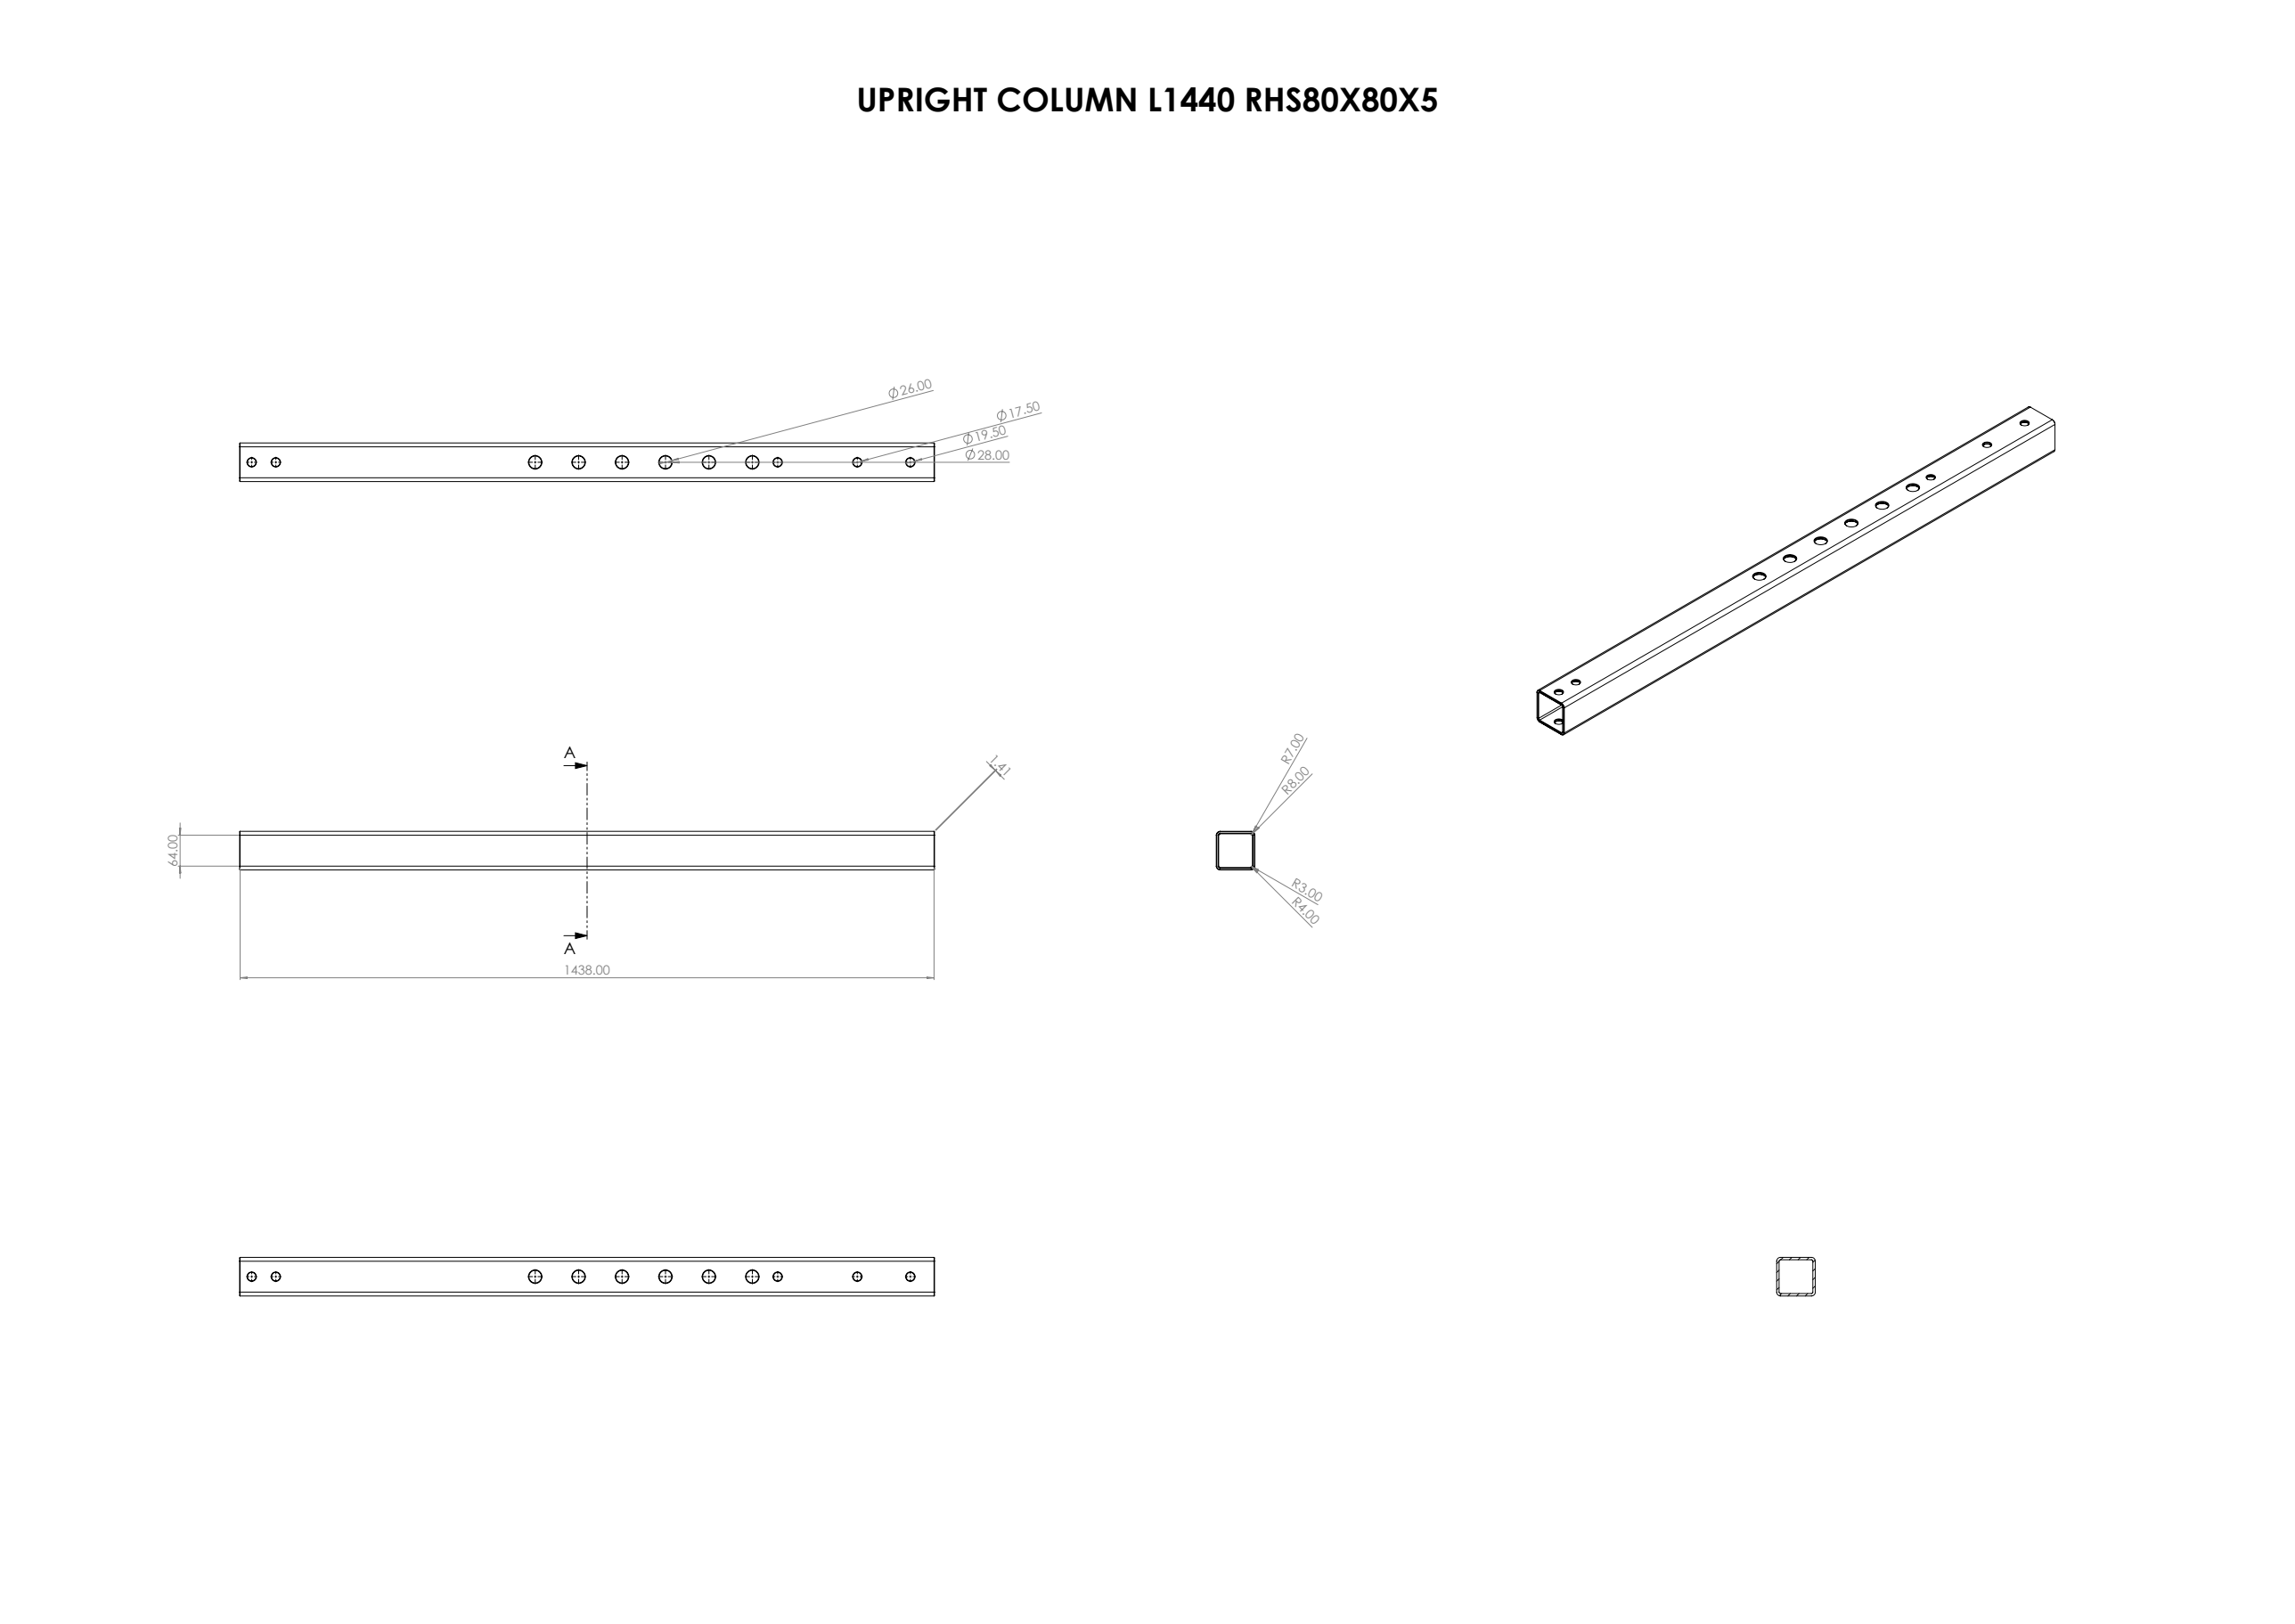
ISO-10303-21;
HEADER;
/* Generated by software containing ST-Developer
 * from STEP Tools, Inc. (www.steptools.com) 
 */

FILE_DESCRIPTION(
/* description */ (''),
/* implementation_level */ '2;1');

FILE_NAME(
/* name */ '01_Upright_Column_L1440_RHS80x80x5.step',
/* time_stamp */ '2026-10-20T10:03:03-07:00',
/* author */ (''),
/* organization */ (''),
/* preprocessor_version */ 'ST-DEVELOPER v20.2',
/* originating_system */ 'Autodesk Translation Framework v15.15.0.0',
/* authorisation */ '');

FILE_SCHEMA (('AUTOMOTIVE_DESIGN { 1 0 10303 214 3 1 1 }'));
ENDSEC;

DATA;
#10=MECHANICAL_DESIGN_GEOMETRIC_PRESENTATION_REPRESENTATION('',(#550),#71492);
#400=SHAPE_REPRESENTATION_RELATIONSHIP('SRR','None',#71621,#419);
#419=ADVANCED_BREP_SHAPE_REPRESENTATION('',(#438),#71491);
#438=MANIFOLD_SOLID_BREP('Upright',#28477);
#550=STYLED_ITEM('',(#71873),#438);
#1844=CYLINDRICAL_SURFACE('',#30568,0.875);
#1845=CYLINDRICAL_SURFACE('',#30572,0.875);
#1846=CYLINDRICAL_SURFACE('',#30576,0.875);
#1847=CYLINDRICAL_SURFACE('',#30580,0.875);
#1848=CYLINDRICAL_SURFACE('',#30584,0.875);
#1849=CYLINDRICAL_SURFACE('',#30588,1.3);
#1850=CYLINDRICAL_SURFACE('',#30592,1.3);
#1851=CYLINDRICAL_SURFACE('',#30608,0.875);
#1852=CYLINDRICAL_SURFACE('',#30612,0.875);
#1853=CYLINDRICAL_SURFACE('',#30616,0.875);
#1854=CYLINDRICAL_SURFACE('',#30620,0.875);
#1855=CYLINDRICAL_SURFACE('',#30624,0.875);
#1856=CYLINDRICAL_SURFACE('',#30642,0.3);
#1857=CYLINDRICAL_SURFACE('',#30645,0.3);
#1858=CYLINDRICAL_SURFACE('',#30654,1.3);
#1859=CYLINDRICAL_SURFACE('',#30658,1.3);
#1860=CYLINDRICAL_SURFACE('',#30662,1.3);
#1861=CYLINDRICAL_SURFACE('',#30666,1.3);
#1862=CYLINDRICAL_SURFACE('',#30670,1.3);
#1863=CYLINDRICAL_SURFACE('',#30674,1.3);
#1864=CYLINDRICAL_SURFACE('',#30678,1.3);
#1865=CYLINDRICAL_SURFACE('',#30682,1.3);
#1866=CYLINDRICAL_SURFACE('',#30686,1.3);
#1867=CYLINDRICAL_SURFACE('',#30707,1.3);
#1868=CYLINDRICAL_SURFACE('',#30738,0.8);
#1869=CYLINDRICAL_SURFACE('',#30741,0.8);
#1870=CYLINDRICAL_SURFACE('',#30769,0.8);
#1871=CYLINDRICAL_SURFACE('',#30785,0.3);
#1872=CYLINDRICAL_SURFACE('',#30786,0.3);
#1873=CYLINDRICAL_SURFACE('',#30789,0.8);
#1999=FACE_BOUND('',#6142,.T.);
#2000=FACE_BOUND('',#6143,.T.);
#2001=FACE_BOUND('',#6144,.T.);
#2002=FACE_BOUND('',#6145,.T.);
#2003=FACE_BOUND('',#6146,.T.);
#2004=FACE_BOUND('',#6147,.T.);
#2005=FACE_BOUND('',#6148,.T.);
#2006=FACE_BOUND('',#6149,.T.);
#2007=FACE_BOUND('',#6150,.T.);
#2008=FACE_BOUND('',#6151,.T.);
#2009=FACE_BOUND('',#6152,.T.);
#2010=FACE_BOUND('',#6168,.T.);
#2011=FACE_BOUND('',#6169,.T.);
#2012=FACE_BOUND('',#6170,.T.);
#2013=FACE_BOUND('',#6171,.T.);
#2014=FACE_BOUND('',#6172,.T.);
#2015=FACE_BOUND('',#6173,.T.);
#2016=FACE_BOUND('',#6174,.T.);
#2017=FACE_BOUND('',#6175,.T.);
#2018=FACE_BOUND('',#6176,.T.);
#2019=FACE_BOUND('',#6177,.T.);
#2020=FACE_BOUND('',#6178,.T.);
#2021=FACE_BOUND('',#6200,.T.);
#2022=FACE_BOUND('',#6221,.T.);
#2023=FACE_BOUND('',#6222,.T.);
#2024=FACE_BOUND('',#6223,.T.);
#2025=FACE_BOUND('',#6224,.T.);
#2026=FACE_BOUND('',#6225,.T.);
#2027=FACE_BOUND('',#6226,.T.);
#2028=FACE_BOUND('',#6227,.T.);
#2029=FACE_BOUND('',#6228,.T.);
#2030=FACE_BOUND('',#6229,.T.);
#2031=FACE_BOUND('',#6230,.T.);
#2032=FACE_BOUND('',#6231,.T.);
#2033=FACE_BOUND('',#6240,.T.);
#2034=FACE_BOUND('',#6241,.T.);
#2035=FACE_BOUND('',#6242,.T.);
#2036=FACE_BOUND('',#6243,.T.);
#2037=FACE_BOUND('',#6244,.T.);
#2038=FACE_BOUND('',#6245,.T.);
#2039=FACE_BOUND('',#6246,.T.);
#2040=FACE_BOUND('',#6247,.T.);
#2041=FACE_BOUND('',#6248,.T.);
#2042=FACE_BOUND('',#6249,.T.);
#2043=FACE_BOUND('',#6250,.T.);
#2044=FACE_BOUND('',#6288,.T.);
#2611=CIRCLE('',#30555,0.975000000000001);
#2612=CIRCLE('',#30556,0.875);
#2613=CIRCLE('',#30558,0.975000000000001);
#2614=CIRCLE('',#30559,0.975000000000001);
#2615=CIRCLE('',#30560,1.4);
#2616=CIRCLE('',#30561,1.4);
#2617=CIRCLE('',#30562,1.4);
#2618=CIRCLE('',#30563,1.4);
#2619=CIRCLE('',#30564,1.4);
#2620=CIRCLE('',#30565,1.4);
#2621=CIRCLE('',#30566,0.975000000000001);
#2622=CIRCLE('',#30567,0.975000000000001);
#2623=CIRCLE('',#30569,0.875);
#2624=CIRCLE('',#30571,0.875);
#2625=CIRCLE('',#30573,0.875);
#2626=CIRCLE('',#30575,0.875);
#2627=CIRCLE('',#30577,0.875);
#2628=CIRCLE('',#30579,0.875);
#2629=CIRCLE('',#30581,0.875);
#2630=CIRCLE('',#30583,0.875);
#2631=CIRCLE('',#30585,0.875);
#2632=CIRCLE('',#30587,1.3);
#2633=CIRCLE('',#30589,1.3);
#2634=CIRCLE('',#30591,1.3);
#2635=CIRCLE('',#30593,1.3);
#2636=CIRCLE('',#30595,0.975000000000001);
#2637=CIRCLE('',#30596,0.875);
#2638=CIRCLE('',#30598,0.975000000000001);
#2639=CIRCLE('',#30599,0.975000000000001);
#2640=CIRCLE('',#30600,1.4);
#2641=CIRCLE('',#30601,1.4);
#2642=CIRCLE('',#30602,1.4);
#2643=CIRCLE('',#30603,1.4);
#2644=CIRCLE('',#30604,1.4);
#2645=CIRCLE('',#30605,1.4);
#2646=CIRCLE('',#30606,0.975000000000001);
#2647=CIRCLE('',#30607,0.975000000000001);
#2648=CIRCLE('',#30609,0.875);
#2649=CIRCLE('',#30611,0.875);
#2650=CIRCLE('',#30613,0.875);
#2651=CIRCLE('',#30615,0.875);
#2652=CIRCLE('',#30617,0.875);
#2653=CIRCLE('',#30619,0.875);
#2654=CIRCLE('',#30621,0.875);
#2655=CIRCLE('',#30623,0.875);
#2656=CIRCLE('',#30625,0.875);
#2657=CIRCLE('',#30628,0.3);
#2658=CIRCLE('',#30629,0.400000000000004);
#2659=CIRCLE('',#30632,0.3);
#2660=CIRCLE('',#30633,0.4);
#2661=CIRCLE('',#30636,0.3);
#2662=CIRCLE('',#30637,0.400000000000003);
#2663=CIRCLE('',#30640,0.3);
#2664=CIRCLE('',#30641,0.400000000000003);
#2665=CIRCLE('',#30643,0.3);
#2666=CIRCLE('',#30646,0.3);
#2667=CIRCLE('',#30648,0.699999999999997);
#2668=CIRCLE('',#30649,0.699999999999997);
#2669=CIRCLE('',#30650,0.7);
#2670=CIRCLE('',#30651,0.700000000000001);
#2671=CIRCLE('',#30653,1.3);
#2672=CIRCLE('',#30655,1.3);
#2673=CIRCLE('',#30657,1.3);
#2674=CIRCLE('',#30659,1.3);
#2675=CIRCLE('',#30661,1.3);
#2676=CIRCLE('',#30663,1.3);
#2677=CIRCLE('',#30665,1.3);
#2678=CIRCLE('',#30667,1.3);
#2679=CIRCLE('',#30669,1.3);
#2680=CIRCLE('',#30671,1.3);
#2681=CIRCLE('',#30673,1.3);
#2682=CIRCLE('',#30675,1.3);
#2683=CIRCLE('',#30677,1.3);
#2684=CIRCLE('',#30679,1.3);
#2685=CIRCLE('',#30681,1.3);
#2686=CIRCLE('',#30683,1.3);
#2687=CIRCLE('',#30685,1.3);
#2688=CIRCLE('',#30687,1.3);
#2689=CIRCLE('',#30689,0.975000000000001);
#2690=CIRCLE('',#30691,0.975000000000001);
#2691=CIRCLE('',#30692,0.975000000000001);
#2692=CIRCLE('',#30693,1.4);
#2693=CIRCLE('',#30694,1.4);
#2694=CIRCLE('',#30695,1.4);
#2695=CIRCLE('',#30696,1.4);
#2696=CIRCLE('',#30697,1.4);
#2697=CIRCLE('',#30698,1.4);
#2698=CIRCLE('',#30699,0.975000000000001);
#2699=CIRCLE('',#30700,0.975000000000001);
#2700=CIRCLE('',#30706,1.3);
#2701=CIRCLE('',#30708,1.3);
#2702=CIRCLE('',#30710,0.975000000000001);
#2703=CIRCLE('',#30712,0.975000000000001);
#2704=CIRCLE('',#30713,0.975000000000001);
#2705=CIRCLE('',#30714,1.4);
#2706=CIRCLE('',#30715,1.4);
#2707=CIRCLE('',#30716,1.4);
#2708=CIRCLE('',#30717,1.4);
#2709=CIRCLE('',#30718,1.4);
#2710=CIRCLE('',#30719,1.4);
#2711=CIRCLE('',#30720,0.975000000000001);
#2712=CIRCLE('',#30721,0.975000000000001);
#2713=CIRCLE('',#30728,0.8);
#2714=CIRCLE('',#30731,0.8);
#2715=CIRCLE('',#30734,0.8);
#2716=CIRCLE('',#30737,0.8);
#2717=CIRCLE('',#30739,0.8);
#2718=CIRCLE('',#30742,0.8);
#2719=CIRCLE('',#30756,0.8);
#2720=CIRCLE('',#30757,0.7);
#2721=CIRCLE('',#30760,0.8);
#2722=CIRCLE('',#30761,0.700000000000001);
#2723=CIRCLE('',#30764,0.699999999999997);
#2724=CIRCLE('',#30767,0.699999999999997);
#2725=CIRCLE('',#30771,0.4);
#2726=CIRCLE('',#30772,0.400000000000003);
#2727=CIRCLE('',#30773,0.400000000000003);
#2728=CIRCLE('',#30774,0.400000000000004);
#2729=CIRCLE('',#30776,0.3);
#2730=CIRCLE('',#30779,0.3);
#2911=CONICAL_SURFACE('',#30554,0.925000000000001,0.785398163397455);
#2912=CONICAL_SURFACE('',#30570,0.925000000000001,0.785398163397455);
#2913=CONICAL_SURFACE('',#30574,0.925000000000001,0.785398163397455);
#2914=CONICAL_SURFACE('',#30578,0.925000000000001,0.785398163397455);
#2915=CONICAL_SURFACE('',#30582,0.925000000000001,0.785398163397455);
#2916=CONICAL_SURFACE('',#30586,1.35,0.785398163397455);
#2917=CONICAL_SURFACE('',#30590,1.35,0.785398163397455);
#2918=CONICAL_SURFACE('',#30594,0.925000000000001,0.785398163397455);
#2919=CONICAL_SURFACE('',#30610,0.925000000000001,0.785398163397455);
#2920=CONICAL_SURFACE('',#30614,0.925000000000001,0.785398163397455);
#2921=CONICAL_SURFACE('',#30618,0.925000000000001,0.785398163397455);
#2922=CONICAL_SURFACE('',#30622,0.925000000000001,0.785398163397455);
#2923=CONICAL_SURFACE('',#30627,0.350000000000002,0.785398163397469);
#2924=CONICAL_SURFACE('',#30631,0.35,0.785398163397446);
#2925=CONICAL_SURFACE('',#30635,0.350000000000001,0.785398163397461);
#2926=CONICAL_SURFACE('',#30639,0.350000000000001,0.785398163397461);
#2927=CONICAL_SURFACE('',#30652,1.35,0.785398163397455);
#2928=CONICAL_SURFACE('',#30656,1.35,0.785398163397455);
#2929=CONICAL_SURFACE('',#30660,1.35,0.785398163397455);
#2930=CONICAL_SURFACE('',#30664,1.35,0.785398163397455);
#2931=CONICAL_SURFACE('',#30668,1.35,0.785398163397455);
#2932=CONICAL_SURFACE('',#30672,1.35,0.785398163397455);
#2933=CONICAL_SURFACE('',#30676,1.35,0.785398163397455);
#2934=CONICAL_SURFACE('',#30680,1.35,0.785398163397455);
#2935=CONICAL_SURFACE('',#30684,1.35,0.785398163397455);
#2936=CONICAL_SURFACE('',#30688,0.925000000000001,0.785398163397455);
#2937=CONICAL_SURFACE('',#30701,0.925000000000001,0.785398163397455);
#2938=CONICAL_SURFACE('',#30702,0.925000000000001,0.785398163397455);
#2939=CONICAL_SURFACE('',#30703,0.925000000000001,0.785398163397455);
#2940=CONICAL_SURFACE('',#30704,0.925000000000001,0.785398163397455);
#2941=CONICAL_SURFACE('',#30705,1.35,0.785398163397455);
#2942=CONICAL_SURFACE('',#30709,0.925000000000001,0.785398163397455);
#2943=CONICAL_SURFACE('',#30722,0.925000000000001,0.785398163397455);
#2944=CONICAL_SURFACE('',#30723,0.925000000000001,0.785398163397455);
#2945=CONICAL_SURFACE('',#30724,0.925000000000001,0.785398163397455);
#2946=CONICAL_SURFACE('',#30725,0.925000000000001,0.785398163397455);
#2947=CONICAL_SURFACE('',#30727,0.75,0.785398163397444);
#2948=CONICAL_SURFACE('',#30730,0.75,0.785398163397447);
#2949=CONICAL_SURFACE('',#30733,0.749999999999998,0.785398163397465);
#2950=CONICAL_SURFACE('',#30736,0.749999999999998,0.785398163397465);
#2951=CONICAL_SURFACE('',#30743,1.35,0.785398163397455);
#2952=CONICAL_SURFACE('',#30744,1.35,0.785398163397455);
#2953=CONICAL_SURFACE('',#30745,1.35,0.785398163397455);
#2954=CONICAL_SURFACE('',#30746,1.35,0.785398163397455);
#2955=CONICAL_SURFACE('',#30747,1.35,0.785398163397455);
#2956=CONICAL_SURFACE('',#30748,1.35,0.785398163397455);
#2957=CONICAL_SURFACE('',#30749,1.35,0.785398163397455);
#2958=CONICAL_SURFACE('',#30750,1.35,0.785398163397455);
#2959=CONICAL_SURFACE('',#30751,1.35,0.785398163397455);
#2960=CONICAL_SURFACE('',#30752,1.35,0.785398163397455);
#2961=CONICAL_SURFACE('',#30753,1.35,0.785398163397455);
#2962=CONICAL_SURFACE('',#30754,1.35,0.785398163397455);
#2963=CONICAL_SURFACE('',#30755,0.75,0.785398163397475);
#2964=CONICAL_SURFACE('',#30759,0.75,0.785398163397472);
#2965=CONICAL_SURFACE('',#30763,0.749999999999998,0.785398163397494);
#2966=CONICAL_SURFACE('',#30766,0.749999999999998,0.785398163397494);
#2967=CONICAL_SURFACE('',#30775,0.35,0.785398163397474);
#2968=CONICAL_SURFACE('',#30778,0.350000000000002,0.785398163397498);
#2969=CONICAL_SURFACE('',#30781,0.350000000000001,0.78539816339749);
#2970=CONICAL_SURFACE('',#30783,0.350000000000001,0.78539816339749);
#4435=FACE_OUTER_BOUND('',#6140,.T.);
#4436=FACE_OUTER_BOUND('',#6141,.T.);
#4437=FACE_OUTER_BOUND('',#6153,.T.);
#4438=FACE_OUTER_BOUND('',#6154,.T.);
#4439=FACE_OUTER_BOUND('',#6155,.T.);
#4440=FACE_OUTER_BOUND('',#6156,.T.);
#4441=FACE_OUTER_BOUND('',#6157,.T.);
#4442=FACE_OUTER_BOUND('',#6158,.T.);
#4443=FACE_OUTER_BOUND('',#6159,.T.);
#4444=FACE_OUTER_BOUND('',#6160,.T.);
#4445=FACE_OUTER_BOUND('',#6161,.T.);
#4446=FACE_OUTER_BOUND('',#6162,.T.);
#4447=FACE_OUTER_BOUND('',#6163,.T.);
#4448=FACE_OUTER_BOUND('',#6164,.T.);
#4449=FACE_OUTER_BOUND('',#6165,.T.);
#4450=FACE_OUTER_BOUND('',#6166,.T.);
#4451=FACE_OUTER_BOUND('',#6167,.T.);
#4452=FACE_OUTER_BOUND('',#6179,.T.);
#4453=FACE_OUTER_BOUND('',#6180,.T.);
#4454=FACE_OUTER_BOUND('',#6181,.T.);
#4455=FACE_OUTER_BOUND('',#6182,.T.);
#4456=FACE_OUTER_BOUND('',#6183,.T.);
#4457=FACE_OUTER_BOUND('',#6184,.T.);
#4458=FACE_OUTER_BOUND('',#6185,.T.);
#4459=FACE_OUTER_BOUND('',#6186,.T.);
#4460=FACE_OUTER_BOUND('',#6187,.T.);
#4461=FACE_OUTER_BOUND('',#6188,.T.);
#4462=FACE_OUTER_BOUND('',#6189,.T.);
#4463=FACE_OUTER_BOUND('',#6190,.T.);
#4464=FACE_OUTER_BOUND('',#6191,.T.);
#4465=FACE_OUTER_BOUND('',#6192,.T.);
#4466=FACE_OUTER_BOUND('',#6193,.T.);
#4467=FACE_OUTER_BOUND('',#6194,.T.);
#4468=FACE_OUTER_BOUND('',#6195,.T.);
#4469=FACE_OUTER_BOUND('',#6196,.T.);
#4470=FACE_OUTER_BOUND('',#6197,.T.);
#4471=FACE_OUTER_BOUND('',#6198,.T.);
#4472=FACE_OUTER_BOUND('',#6199,.T.);
#4473=FACE_OUTER_BOUND('',#6201,.T.);
#4474=FACE_OUTER_BOUND('',#6202,.T.);
#4475=FACE_OUTER_BOUND('',#6203,.T.);
#4476=FACE_OUTER_BOUND('',#6204,.T.);
#4477=FACE_OUTER_BOUND('',#6205,.T.);
#4478=FACE_OUTER_BOUND('',#6206,.T.);
#4479=FACE_OUTER_BOUND('',#6207,.T.);
#4480=FACE_OUTER_BOUND('',#6208,.T.);
#4481=FACE_OUTER_BOUND('',#6209,.T.);
#4482=FACE_OUTER_BOUND('',#6210,.T.);
#4483=FACE_OUTER_BOUND('',#6211,.T.);
#4484=FACE_OUTER_BOUND('',#6212,.T.);
#4485=FACE_OUTER_BOUND('',#6213,.T.);
#4486=FACE_OUTER_BOUND('',#6214,.T.);
#4487=FACE_OUTER_BOUND('',#6215,.T.);
#4488=FACE_OUTER_BOUND('',#6216,.T.);
#4489=FACE_OUTER_BOUND('',#6217,.T.);
#4490=FACE_OUTER_BOUND('',#6218,.T.);
#4491=FACE_OUTER_BOUND('',#6219,.T.);
#4492=FACE_OUTER_BOUND('',#6220,.T.);
#4493=FACE_OUTER_BOUND('',#6232,.T.);
#4494=FACE_OUTER_BOUND('',#6233,.T.);
#4495=FACE_OUTER_BOUND('',#6234,.T.);
#4496=FACE_OUTER_BOUND('',#6235,.T.);
#4497=FACE_OUTER_BOUND('',#6236,.T.);
#4498=FACE_OUTER_BOUND('',#6237,.T.);
#4499=FACE_OUTER_BOUND('',#6238,.T.);
#4500=FACE_OUTER_BOUND('',#6239,.T.);
#4501=FACE_OUTER_BOUND('',#6251,.T.);
#4502=FACE_OUTER_BOUND('',#6252,.T.);
#4503=FACE_OUTER_BOUND('',#6253,.T.);
#4504=FACE_OUTER_BOUND('',#6254,.T.);
#4505=FACE_OUTER_BOUND('',#6255,.T.);
#4506=FACE_OUTER_BOUND('',#6256,.T.);
#4507=FACE_OUTER_BOUND('',#6257,.T.);
#4508=FACE_OUTER_BOUND('',#6258,.T.);
#4509=FACE_OUTER_BOUND('',#6259,.T.);
#4510=FACE_OUTER_BOUND('',#6260,.T.);
#4511=FACE_OUTER_BOUND('',#6261,.T.);
#4512=FACE_OUTER_BOUND('',#6262,.T.);
#4513=FACE_OUTER_BOUND('',#6263,.T.);
#4514=FACE_OUTER_BOUND('',#6264,.T.);
#4515=FACE_OUTER_BOUND('',#6265,.T.);
#4516=FACE_OUTER_BOUND('',#6266,.T.);
#4517=FACE_OUTER_BOUND('',#6267,.T.);
#4518=FACE_OUTER_BOUND('',#6268,.T.);
#4519=FACE_OUTER_BOUND('',#6269,.T.);
#4520=FACE_OUTER_BOUND('',#6270,.T.);
#4521=FACE_OUTER_BOUND('',#6271,.T.);
#4522=FACE_OUTER_BOUND('',#6272,.T.);
#4523=FACE_OUTER_BOUND('',#6273,.T.);
#4524=FACE_OUTER_BOUND('',#6274,.T.);
#4525=FACE_OUTER_BOUND('',#6275,.T.);
#4526=FACE_OUTER_BOUND('',#6276,.T.);
#4527=FACE_OUTER_BOUND('',#6277,.T.);
#4528=FACE_OUTER_BOUND('',#6278,.T.);
#4529=FACE_OUTER_BOUND('',#6279,.T.);
#4530=FACE_OUTER_BOUND('',#6280,.T.);
#4531=FACE_OUTER_BOUND('',#6281,.T.);
#4532=FACE_OUTER_BOUND('',#6282,.T.);
#4533=FACE_OUTER_BOUND('',#6283,.T.);
#4534=FACE_OUTER_BOUND('',#6284,.T.);
#4535=FACE_OUTER_BOUND('',#6285,.T.);
#4536=FACE_OUTER_BOUND('',#6286,.T.);
#4537=FACE_OUTER_BOUND('',#6287,.T.);
#4538=FACE_OUTER_BOUND('',#6289,.T.);
#4539=FACE_OUTER_BOUND('',#6290,.T.);
#4540=FACE_OUTER_BOUND('',#6291,.T.);
#4541=FACE_OUTER_BOUND('',#6292,.T.);
#4542=FACE_OUTER_BOUND('',#6293,.T.);
#4543=FACE_OUTER_BOUND('',#6294,.T.);
#4544=FACE_OUTER_BOUND('',#6295,.T.);
#4545=FACE_OUTER_BOUND('',#6296,.T.);
#4546=FACE_OUTER_BOUND('',#6297,.T.);
#4547=FACE_OUTER_BOUND('',#6298,.T.);
#4548=FACE_OUTER_BOUND('',#6299,.T.);
#4549=FACE_OUTER_BOUND('',#6300,.T.);
#4550=FACE_OUTER_BOUND('',#6301,.T.);
#6140=EDGE_LOOP('',(#25539,#25540,#25541,#25542));
#6141=EDGE_LOOP('',(#25543,#25544,#25545,#25546));
#6142=EDGE_LOOP('',(#25547));
#6143=EDGE_LOOP('',(#25548));
#6144=EDGE_LOOP('',(#25549));
#6145=EDGE_LOOP('',(#25550));
#6146=EDGE_LOOP('',(#25551));
#6147=EDGE_LOOP('',(#25552));
#6148=EDGE_LOOP('',(#25553));
#6149=EDGE_LOOP('',(#25554));
#6150=EDGE_LOOP('',(#25555));
#6151=EDGE_LOOP('',(#25556));
#6152=EDGE_LOOP('',(#25557));
#6153=EDGE_LOOP('',(#25558,#25559,#25560,#25561));
#6154=EDGE_LOOP('',(#25562,#25563,#25564,#25565));
#6155=EDGE_LOOP('',(#25566,#25567,#25568,#25569));
#6156=EDGE_LOOP('',(#25570,#25571,#25572,#25573));
#6157=EDGE_LOOP('',(#25574,#25575,#25576,#25577));
#6158=EDGE_LOOP('',(#25578,#25579,#25580,#25581));
#6159=EDGE_LOOP('',(#25582,#25583,#25584,#25585));
#6160=EDGE_LOOP('',(#25586,#25587,#25588,#25589));
#6161=EDGE_LOOP('',(#25590,#25591,#25592,#25593));
#6162=EDGE_LOOP('',(#25594,#25595,#25596,#25597));
#6163=EDGE_LOOP('',(#25598,#25599,#25600,#25601));
#6164=EDGE_LOOP('',(#25602,#25603,#25604,#25605));
#6165=EDGE_LOOP('',(#25606,#25607,#25608,#25609));
#6166=EDGE_LOOP('',(#25610,#25611,#25612,#25613));
#6167=EDGE_LOOP('',(#25614,#25615,#25616,#25617));
#6168=EDGE_LOOP('',(#25618));
#6169=EDGE_LOOP('',(#25619));
#6170=EDGE_LOOP('',(#25620));
#6171=EDGE_LOOP('',(#25621));
#6172=EDGE_LOOP('',(#25622));
#6173=EDGE_LOOP('',(#25623));
#6174=EDGE_LOOP('',(#25624));
#6175=EDGE_LOOP('',(#25625));
#6176=EDGE_LOOP('',(#25626));
#6177=EDGE_LOOP('',(#25627));
#6178=EDGE_LOOP('',(#25628));
#6179=EDGE_LOOP('',(#25629,#25630,#25631,#25632));
#6180=EDGE_LOOP('',(#25633,#25634,#25635,#25636));
#6181=EDGE_LOOP('',(#25637,#25638,#25639,#25640));
#6182=EDGE_LOOP('',(#25641,#25642,#25643,#25644));
#6183=EDGE_LOOP('',(#25645,#25646,#25647,#25648));
#6184=EDGE_LOOP('',(#25649,#25650,#25651,#25652));
#6185=EDGE_LOOP('',(#25653,#25654,#25655,#25656));
#6186=EDGE_LOOP('',(#25657,#25658,#25659,#25660));
#6187=EDGE_LOOP('',(#25661,#25662,#25663,#25664));
#6188=EDGE_LOOP('',(#25665,#25666,#25667,#25668));
#6189=EDGE_LOOP('',(#25669,#25670,#25671,#25672));
#6190=EDGE_LOOP('',(#25673,#25674,#25675,#25676));
#6191=EDGE_LOOP('',(#25677,#25678,#25679,#25680));
#6192=EDGE_LOOP('',(#25681,#25682,#25683,#25684));
#6193=EDGE_LOOP('',(#25685,#25686,#25687,#25688));
#6194=EDGE_LOOP('',(#25689,#25690,#25691,#25692));
#6195=EDGE_LOOP('',(#25693,#25694,#25695,#25696));
#6196=EDGE_LOOP('',(#25697,#25698,#25699,#25700));
#6197=EDGE_LOOP('',(#25701,#25702,#25703,#25704));
#6198=EDGE_LOOP('',(#25705,#25706,#25707,#25708));
#6199=EDGE_LOOP('',(#25709,#25710,#25711,#25712,#25713,#25714,#25715,#25716));
#6200=EDGE_LOOP('',(#25717,#25718,#25719,#25720,#25721,#25722,#25723,#25724));
#6201=EDGE_LOOP('',(#25725,#25726,#25727,#25728));
#6202=EDGE_LOOP('',(#25729,#25730,#25731,#25732));
#6203=EDGE_LOOP('',(#25733,#25734,#25735,#25736));
#6204=EDGE_LOOP('',(#25737,#25738,#25739,#25740));
#6205=EDGE_LOOP('',(#25741,#25742,#25743,#25744));
#6206=EDGE_LOOP('',(#25745,#25746,#25747,#25748));
#6207=EDGE_LOOP('',(#25749,#25750,#25751,#25752));
#6208=EDGE_LOOP('',(#25753,#25754,#25755,#25756));
#6209=EDGE_LOOP('',(#25757,#25758,#25759,#25760));
#6210=EDGE_LOOP('',(#25761,#25762,#25763,#25764));
#6211=EDGE_LOOP('',(#25765,#25766,#25767,#25768));
#6212=EDGE_LOOP('',(#25769,#25770,#25771,#25772));
#6213=EDGE_LOOP('',(#25773,#25774,#25775,#25776));
#6214=EDGE_LOOP('',(#25777,#25778,#25779,#25780));
#6215=EDGE_LOOP('',(#25781,#25782,#25783,#25784));
#6216=EDGE_LOOP('',(#25785,#25786,#25787,#25788));
#6217=EDGE_LOOP('',(#25789,#25790,#25791,#25792));
#6218=EDGE_LOOP('',(#25793,#25794,#25795,#25796));
#6219=EDGE_LOOP('',(#25797,#25798,#25799,#25800));
#6220=EDGE_LOOP('',(#25801,#25802,#25803,#25804));
#6221=EDGE_LOOP('',(#25805));
#6222=EDGE_LOOP('',(#25806));
#6223=EDGE_LOOP('',(#25807));
#6224=EDGE_LOOP('',(#25808));
#6225=EDGE_LOOP('',(#25809));
#6226=EDGE_LOOP('',(#25810));
#6227=EDGE_LOOP('',(#25811));
#6228=EDGE_LOOP('',(#25812));
#6229=EDGE_LOOP('',(#25813));
#6230=EDGE_LOOP('',(#25814));
#6231=EDGE_LOOP('',(#25815));
#6232=EDGE_LOOP('',(#25816,#25817,#25818,#25819));
#6233=EDGE_LOOP('',(#25820,#25821,#25822,#25823));
#6234=EDGE_LOOP('',(#25824,#25825,#25826,#25827));
#6235=EDGE_LOOP('',(#25828,#25829,#25830,#25831));
#6236=EDGE_LOOP('',(#25832,#25833,#25834,#25835));
#6237=EDGE_LOOP('',(#25836,#25837,#25838,#25839));
#6238=EDGE_LOOP('',(#25840,#25841,#25842,#25843));
#6239=EDGE_LOOP('',(#25844,#25845,#25846,#25847));
#6240=EDGE_LOOP('',(#25848));
#6241=EDGE_LOOP('',(#25849));
#6242=EDGE_LOOP('',(#25850));
#6243=EDGE_LOOP('',(#25851));
#6244=EDGE_LOOP('',(#25852));
#6245=EDGE_LOOP('',(#25853));
#6246=EDGE_LOOP('',(#25854));
#6247=EDGE_LOOP('',(#25855));
#6248=EDGE_LOOP('',(#25856));
#6249=EDGE_LOOP('',(#25857));
#6250=EDGE_LOOP('',(#25858));
#6251=EDGE_LOOP('',(#25859,#25860,#25861,#25862));
#6252=EDGE_LOOP('',(#25863,#25864,#25865,#25866));
#6253=EDGE_LOOP('',(#25867,#25868,#25869,#25870));
#6254=EDGE_LOOP('',(#25871,#25872,#25873,#25874));
#6255=EDGE_LOOP('',(#25875,#25876,#25877,#25878));
#6256=EDGE_LOOP('',(#25879,#25880,#25881,#25882));
#6257=EDGE_LOOP('',(#25883,#25884,#25885,#25886));
#6258=EDGE_LOOP('',(#25887,#25888,#25889,#25890));
#6259=EDGE_LOOP('',(#25891,#25892,#25893,#25894));
#6260=EDGE_LOOP('',(#25895,#25896,#25897,#25898));
#6261=EDGE_LOOP('',(#25899,#25900,#25901,#25902));
#6262=EDGE_LOOP('',(#25903,#25904,#25905,#25906));
#6263=EDGE_LOOP('',(#25907,#25908,#25909,#25910));
#6264=EDGE_LOOP('',(#25911,#25912,#25913,#25914));
#6265=EDGE_LOOP('',(#25915,#25916,#25917,#25918));
#6266=EDGE_LOOP('',(#25919,#25920,#25921,#25922));
#6267=EDGE_LOOP('',(#25923,#25924,#25925,#25926));
#6268=EDGE_LOOP('',(#25927,#25928,#25929,#25930));
#6269=EDGE_LOOP('',(#25931,#25932,#25933,#25934));
#6270=EDGE_LOOP('',(#25935,#25936,#25937,#25938));
#6271=EDGE_LOOP('',(#25939,#25940,#25941,#25942));
#6272=EDGE_LOOP('',(#25943,#25944,#25945,#25946));
#6273=EDGE_LOOP('',(#25947,#25948,#25949,#25950));
#6274=EDGE_LOOP('',(#25951,#25952,#25953,#25954));
#6275=EDGE_LOOP('',(#25955,#25956,#25957,#25958));
#6276=EDGE_LOOP('',(#25959,#25960,#25961,#25962));
#6277=EDGE_LOOP('',(#25963,#25964,#25965,#25966));
#6278=EDGE_LOOP('',(#25967,#25968,#25969,#25970));
#6279=EDGE_LOOP('',(#25971,#25972,#25973,#25974));
#6280=EDGE_LOOP('',(#25975,#25976,#25977,#25978));
#6281=EDGE_LOOP('',(#25979,#25980,#25981,#25982));
#6282=EDGE_LOOP('',(#25983,#25984,#25985,#25986));
#6283=EDGE_LOOP('',(#25987,#25988,#25989,#25990));
#6284=EDGE_LOOP('',(#25991,#25992,#25993,#25994));
#6285=EDGE_LOOP('',(#25995,#25996,#25997,#25998));
#6286=EDGE_LOOP('',(#25999,#26000,#26001,#26002));
#6287=EDGE_LOOP('',(#26003,#26004,#26005,#26006,#26007,#26008,#26009,#26010));
#6288=EDGE_LOOP('',(#26011,#26012,#26013,#26014,#26015,#26016,#26017,#26018));
#6289=EDGE_LOOP('',(#26019,#26020,#26021,#26022));
#6290=EDGE_LOOP('',(#26023,#26024,#26025,#26026));
#6291=EDGE_LOOP('',(#26027,#26028,#26029,#26030));
#6292=EDGE_LOOP('',(#26031,#26032,#26033,#26034));
#6293=EDGE_LOOP('',(#26035,#26036,#26037,#26038));
#6294=EDGE_LOOP('',(#26039,#26040,#26041,#26042));
#6295=EDGE_LOOP('',(#26043,#26044,#26045,#26046));
#6296=EDGE_LOOP('',(#26047,#26048,#26049,#26050));
#6297=EDGE_LOOP('',(#26051,#26052,#26053,#26054));
#6298=EDGE_LOOP('',(#26055,#26056,#26057,#26058));
#6299=EDGE_LOOP('',(#26059,#26060,#26061,#26062));
#6300=EDGE_LOOP('',(#26063,#26064,#26065,#26066));
#6301=EDGE_LOOP('',(#26067,#26068,#26069,#26070));
#8644=LINE('',#70856,#11132);
#8645=LINE('',#70861,#11133);
#8646=LINE('',#70863,#11134);
#8647=LINE('',#70865,#11135);
#8648=LINE('',#70866,#11136);
#8649=LINE('',#70889,#11137);
#8650=LINE('',#70893,#11138);
#8651=LINE('',#70897,#11139);
#8652=LINE('',#70901,#11140);
#8653=LINE('',#70905,#11141);
#8654=LINE('',#70909,#11142);
#8655=LINE('',#70913,#11143);
#8656=LINE('',#70917,#11144);
#8657=LINE('',#70921,#11145);
#8658=LINE('',#70925,#11146);
#8659=LINE('',#70929,#11147);
#8660=LINE('',#70933,#11148);
#8661=LINE('',#70937,#11149);
#8662=LINE('',#70943,#11150);
#8663=LINE('',#70948,#11151);
#8664=LINE('',#70950,#11152);
#8665=LINE('',#70952,#11153);
#8666=LINE('',#70953,#11154);
#8667=LINE('',#70977,#11155);
#8668=LINE('',#70980,#11156);
#8669=LINE('',#70985,#11157);
#8670=LINE('',#70988,#11158);
#8671=LINE('',#70993,#11159);
#8672=LINE('',#70996,#11160);
#8673=LINE('',#71001,#11161);
#8674=LINE('',#71004,#11162);
#8675=LINE('',#71009,#11163);
#8676=LINE('',#71012,#11164);
#8677=LINE('',#71014,#11165);
#8678=LINE('',#71015,#11166);
#8679=LINE('',#71019,#11167);
#8680=LINE('',#71025,#11168);
#8681=LINE('',#71026,#11169);
#8682=LINE('',#71027,#11170);
#8683=LINE('',#71030,#11171);
#8684=LINE('',#71035,#11172);
#8685=LINE('',#71036,#11173);
#8686=LINE('',#71040,#11174);
#8687=LINE('',#71046,#11175);
#8688=LINE('',#71047,#11176);
#8689=LINE('',#71048,#11177);
#8690=LINE('',#71054,#11178);
#8691=LINE('',#71058,#11179);
#8692=LINE('',#71059,#11180);
#8693=LINE('',#71065,#11181);
#8694=LINE('',#71069,#11182);
#8695=LINE('',#71073,#11183);
#8696=LINE('',#71077,#11184);
#8697=LINE('',#71081,#11185);
#8698=LINE('',#71086,#11186);
#8699=LINE('',#71089,#11187);
#8700=LINE('',#71094,#11188);
#8701=LINE('',#71097,#11189);
#8702=LINE('',#71102,#11190);
#8703=LINE('',#71105,#11191);
#8704=LINE('',#71109,#11192);
#8705=LINE('',#71113,#11193);
#8706=LINE('',#71118,#11194);
#8707=LINE('',#71121,#11195);
#8708=LINE('',#71125,#11196);
#8709=LINE('',#71129,#11197);
#8710=LINE('',#71134,#11198);
#8711=LINE('',#71137,#11199);
#8712=LINE('',#71141,#11200);
#8713=LINE('',#71145,#11201);
#8714=LINE('',#71150,#11202);
#8715=LINE('',#71154,#11203);
#8716=LINE('',#71158,#11204);
#8717=LINE('',#71160,#11205);
#8718=LINE('',#71162,#11206);
#8719=LINE('',#71163,#11207);
#8720=LINE('',#71185,#11208);
#8721=LINE('',#71187,#11209);
#8722=LINE('',#71189,#11210);
#8723=LINE('',#71191,#11211);
#8724=LINE('',#71194,#11212);
#8725=LINE('',#71198,#11213);
#8726=LINE('',#71203,#11214);
#8727=LINE('',#71207,#11215);
#8728=LINE('',#71209,#11216);
#8729=LINE('',#71211,#11217);
#8730=LINE('',#71212,#11218);
#8731=LINE('',#71234,#11219);
#8732=LINE('',#71236,#11220);
#8733=LINE('',#71238,#11221);
#8734=LINE('',#71240,#11222);
#8735=LINE('',#71242,#11223);
#8736=LINE('',#71243,#11224);
#8737=LINE('',#71246,#11225);
#8738=LINE('',#71250,#11226);
#8739=LINE('',#71251,#11227);
#8740=LINE('',#71253,#11228);
#8741=LINE('',#71256,#11229);
#8742=LINE('',#71259,#11230);
#8743=LINE('',#71263,#11231);
#8744=LINE('',#71264,#11232);
#8745=LINE('',#71269,#11233);
#8746=LINE('',#71273,#11234);
#8747=LINE('',#71274,#11235);
#8748=LINE('',#71278,#11236);
#8749=LINE('',#71280,#11237);
#8750=LINE('',#71282,#11238);
#8751=LINE('',#71284,#11239);
#8752=LINE('',#71286,#11240);
#8753=LINE('',#71288,#11241);
#8754=LINE('',#71290,#11242);
#8755=LINE('',#71292,#11243);
#8756=LINE('',#71294,#11244);
#8757=LINE('',#71296,#11245);
#8758=LINE('',#71298,#11246);
#8759=LINE('',#71300,#11247);
#8760=LINE('',#71304,#11248);
#8761=LINE('',#71307,#11249);
#8762=LINE('',#71311,#11250);
#8763=LINE('',#71313,#11251);
#8764=LINE('',#71314,#11252);
#8765=LINE('',#71317,#11253);
#8766=LINE('',#71322,#11254);
#8767=LINE('',#71323,#11255);
#8768=LINE('',#71326,#11256);
#8769=LINE('',#71330,#11257);
#8770=LINE('',#71331,#11258);
#8771=LINE('',#71334,#11259);
#8772=LINE('',#71337,#11260);
#8773=LINE('',#71339,#11261);
#8774=LINE('',#71345,#11262);
#8775=LINE('',#71349,#11263);
#8776=LINE('',#71353,#11264);
#8777=LINE('',#71356,#11265);
#8778=LINE('',#71359,#11266);
#8779=LINE('',#71361,#11267);
#8780=LINE('',#71364,#11268);
#8781=LINE('',#71365,#11269);
#8782=LINE('',#71367,#11270);
#8783=LINE('',#71370,#11271);
#8784=LINE('',#71372,#11272);
#8785=LINE('',#71374,#11273);
#8786=LINE('',#71376,#11274);
#8787=LINE('',#71379,#11275);
#8788=LINE('',#71381,#11276);
#8789=LINE('',#71384,#11277);
#11132=VECTOR('',#36933,0.925000000000001);
#11133=VECTOR('',#36938,1.);
#11134=VECTOR('',#36939,1.);
#11135=VECTOR('',#36940,1.);
#11136=VECTOR('',#36941,1.);
#11137=VECTOR('',#36964,0.875);
#11138=VECTOR('',#36969,0.925000000000001);
#11139=VECTOR('',#36974,0.875);
#11140=VECTOR('',#36979,0.925000000000001);
#11141=VECTOR('',#36984,0.875);
#11142=VECTOR('',#36989,0.925000000000001);
#11143=VECTOR('',#36994,0.875);
#11144=VECTOR('',#36999,0.925);
#11145=VECTOR('',#37004,0.875);
#11146=VECTOR('',#37009,1.35);
#11147=VECTOR('',#37014,1.3);
#11148=VECTOR('',#37019,1.35);
#11149=VECTOR('',#37024,1.3);
#11150=VECTOR('',#37031,0.925000000000001);
#11151=VECTOR('',#37036,1.);
#11152=VECTOR('',#37037,1.);
#11153=VECTOR('',#37038,1.);
#11154=VECTOR('',#37039,1.);
#11155=VECTOR('',#37064,0.875);
#11156=VECTOR('',#37067,0.925000000000001);
#11157=VECTOR('',#37074,0.875);
#11158=VECTOR('',#37077,0.925000000000001);
#11159=VECTOR('',#37084,0.875);
#11160=VECTOR('',#37087,0.925000000000001);
#11161=VECTOR('',#37094,0.875);
#11162=VECTOR('',#37097,0.925);
#11163=VECTOR('',#37104,0.875);
#11164=VECTOR('',#37107,1.);
#11165=VECTOR('',#37108,1.);
#11166=VECTOR('',#37109,1.);
#11167=VECTOR('',#37112,1.);
#11168=VECTOR('',#37119,1.);
#11169=VECTOR('',#37120,1.);
#11170=VECTOR('',#37121,1.);
#11171=VECTOR('',#37124,1.);
#11172=VECTOR('',#37131,1.);
#11173=VECTOR('',#37132,1.);
#11174=VECTOR('',#37135,1.);
#11175=VECTOR('',#37142,1.);
#11176=VECTOR('',#37143,1.);
#11177=VECTOR('',#37144,1.);
#11178=VECTOR('',#37153,1.);
#11179=VECTOR('',#37158,1.);
#11180=VECTOR('',#37159,1.);
#11181=VECTOR('',#37166,1.);
#11182=VECTOR('',#37169,1.);
#11183=VECTOR('',#37172,1.);
#11184=VECTOR('',#37175,1.);
#11185=VECTOR('',#37180,1.35);
#11186=VECTOR('',#37187,1.3);
#11187=VECTOR('',#37190,1.35);
#11188=VECTOR('',#37197,1.3);
#11189=VECTOR('',#37200,1.35);
#11190=VECTOR('',#37207,1.3);
#11191=VECTOR('',#37210,1.35);
#11192=VECTOR('',#37215,1.3);
#11193=VECTOR('',#37220,1.35);
#11194=VECTOR('',#37227,1.3);
#11195=VECTOR('',#37230,1.35);
#11196=VECTOR('',#37235,1.3);
#11197=VECTOR('',#37240,1.35);
#11198=VECTOR('',#37247,1.3);
#11199=VECTOR('',#37250,1.35);
#11200=VECTOR('',#37255,1.3);
#11201=VECTOR('',#37260,1.35);
#11202=VECTOR('',#37267,1.3);
#11203=VECTOR('',#37272,0.925000000000001);
#11204=VECTOR('',#37275,1.);
#11205=VECTOR('',#37276,1.);
#11206=VECTOR('',#37277,1.);
#11207=VECTOR('',#37278,1.);
#11208=VECTOR('',#37301,0.925000000000001);
#11209=VECTOR('',#37304,0.925000000000001);
#11210=VECTOR('',#37307,0.925000000000001);
#11211=VECTOR('',#37310,0.925);
#11212=VECTOR('',#37313,1.35);
#11213=VECTOR('',#37318,1.3);
#11214=VECTOR('',#37325,0.925000000000001);
#11215=VECTOR('',#37328,1.);
#11216=VECTOR('',#37329,1.);
#11217=VECTOR('',#37330,1.);
#11218=VECTOR('',#37331,1.);
#11219=VECTOR('',#37354,0.925000000000001);
#11220=VECTOR('',#37357,0.925000000000001);
#11221=VECTOR('',#37360,0.925000000000001);
#11222=VECTOR('',#37363,0.925);
#11223=VECTOR('',#37366,1.);
#11224=VECTOR('',#37367,1.);
#11225=VECTOR('',#37370,1.);
#11226=VECTOR('',#37375,1.);
#11227=VECTOR('',#37376,1.);
#11228=VECTOR('',#37379,1.);
#11229=VECTOR('',#37384,1.);
#11230=VECTOR('',#37387,1.);
#11231=VECTOR('',#37392,1.);
#11232=VECTOR('',#37393,1.);
#11233=VECTOR('',#37400,1.);
#11234=VECTOR('',#37405,1.);
#11235=VECTOR('',#37406,1.);
#11236=VECTOR('',#37413,1.35);
#11237=VECTOR('',#37416,1.35);
#11238=VECTOR('',#37419,1.35);
#11239=VECTOR('',#37422,1.35);
#11240=VECTOR('',#37425,1.35);
#11241=VECTOR('',#37428,1.35);
#11242=VECTOR('',#37431,1.35);
#11243=VECTOR('',#37434,1.35);
#11244=VECTOR('',#37437,1.35);
#11245=VECTOR('',#37440,1.35);
#11246=VECTOR('',#37443,1.35);
#11247=VECTOR('',#37446,1.35);
#11248=VECTOR('',#37449,1.);
#11249=VECTOR('',#37452,1.);
#11250=VECTOR('',#37457,1.);
#11251=VECTOR('',#37458,1.);
#11252=VECTOR('',#37459,1.);
#11253=VECTOR('',#37462,1.);
#11254=VECTOR('',#37469,1.);
#11255=VECTOR('',#37470,1.);
#11256=VECTOR('',#37473,1.);
#11257=VECTOR('',#37478,1.);
#11258=VECTOR('',#37479,1.);
#11259=VECTOR('',#37482,1.);
#11260=VECTOR('',#37487,1.);
#11261=VECTOR('',#37490,1.);
#11262=VECTOR('',#37495,1.);
#11263=VECTOR('',#37498,1.);
#11264=VECTOR('',#37501,1.);
#11265=VECTOR('',#37504,1.);
#11266=VECTOR('',#37507,1.);
#11267=VECTOR('',#37510,1.);
#11268=VECTOR('',#37513,1.);
#11269=VECTOR('',#37514,1.);
#11270=VECTOR('',#37517,1.);
#11271=VECTOR('',#37522,1.);
#11272=VECTOR('',#37525,1.);
#11273=VECTOR('',#37528,1.);
#11274=VECTOR('',#37531,1.);
#11275=VECTOR('',#37536,1.);
#11276=VECTOR('',#37539,1.);
#11277=VECTOR('',#37544,1.);
#13691=VERTEX_POINT('',#70853);
#13692=VERTEX_POINT('',#70855);
#13693=VERTEX_POINT('',#70859);
#13694=VERTEX_POINT('',#70860);
#13695=VERTEX_POINT('',#70862);
#13696=VERTEX_POINT('',#70864);
#13697=VERTEX_POINT('',#70867);
#13698=VERTEX_POINT('',#70869);
#13699=VERTEX_POINT('',#70871);
#13700=VERTEX_POINT('',#70873);
#13701=VERTEX_POINT('',#70875);
#13702=VERTEX_POINT('',#70877);
#13703=VERTEX_POINT('',#70879);
#13704=VERTEX_POINT('',#70881);
#13705=VERTEX_POINT('',#70883);
#13706=VERTEX_POINT('',#70885);
#13707=VERTEX_POINT('',#70888);
#13708=VERTEX_POINT('',#70892);
#13709=VERTEX_POINT('',#70896);
#13710=VERTEX_POINT('',#70900);
#13711=VERTEX_POINT('',#70904);
#13712=VERTEX_POINT('',#70908);
#13713=VERTEX_POINT('',#70912);
#13714=VERTEX_POINT('',#70916);
#13715=VERTEX_POINT('',#70920);
#13716=VERTEX_POINT('',#70924);
#13717=VERTEX_POINT('',#70928);
#13718=VERTEX_POINT('',#70932);
#13719=VERTEX_POINT('',#70936);
#13720=VERTEX_POINT('',#70940);
#13721=VERTEX_POINT('',#70942);
#13722=VERTEX_POINT('',#70946);
#13723=VERTEX_POINT('',#70947);
#13724=VERTEX_POINT('',#70949);
#13725=VERTEX_POINT('',#70951);
#13726=VERTEX_POINT('',#70954);
#13727=VERTEX_POINT('',#70956);
#13728=VERTEX_POINT('',#70958);
#13729=VERTEX_POINT('',#70960);
#13730=VERTEX_POINT('',#70962);
#13731=VERTEX_POINT('',#70964);
#13732=VERTEX_POINT('',#70966);
#13733=VERTEX_POINT('',#70968);
#13734=VERTEX_POINT('',#70970);
#13735=VERTEX_POINT('',#70972);
#13736=VERTEX_POINT('',#70975);
#13737=VERTEX_POINT('',#70979);
#13738=VERTEX_POINT('',#70983);
#13739=VERTEX_POINT('',#70987);
#13740=VERTEX_POINT('',#70991);
#13741=VERTEX_POINT('',#70995);
#13742=VERTEX_POINT('',#70999);
#13743=VERTEX_POINT('',#71003);
#13744=VERTEX_POINT('',#71007);
#13745=VERTEX_POINT('',#71011);
#13746=VERTEX_POINT('',#71013);
#13747=VERTEX_POINT('',#71017);
#13748=VERTEX_POINT('',#71018);
#13749=VERTEX_POINT('',#71023);
#13750=VERTEX_POINT('',#71024);
#13751=VERTEX_POINT('',#71029);
#13752=VERTEX_POINT('',#71034);
#13753=VERTEX_POINT('',#71038);
#13754=VERTEX_POINT('',#71039);
#13755=VERTEX_POINT('',#71044);
#13756=VERTEX_POINT('',#71045);
#13757=VERTEX_POINT('',#71053);
#13758=VERTEX_POINT('',#71057);
#13759=VERTEX_POINT('',#71063);
#13760=VERTEX_POINT('',#71064);
#13761=VERTEX_POINT('',#71066);
#13762=VERTEX_POINT('',#71068);
#13763=VERTEX_POINT('',#71070);
#13764=VERTEX_POINT('',#71072);
#13765=VERTEX_POINT('',#71074);
#13766=VERTEX_POINT('',#71076);
#13767=VERTEX_POINT('',#71080);
#13768=VERTEX_POINT('',#71084);
#13769=VERTEX_POINT('',#71088);
#13770=VERTEX_POINT('',#71092);
#13771=VERTEX_POINT('',#71096);
#13772=VERTEX_POINT('',#71100);
#13773=VERTEX_POINT('',#71104);
#13774=VERTEX_POINT('',#71108);
#13775=VERTEX_POINT('',#71112);
#13776=VERTEX_POINT('',#71116);
#13777=VERTEX_POINT('',#71120);
#13778=VERTEX_POINT('',#71124);
#13779=VERTEX_POINT('',#71128);
#13780=VERTEX_POINT('',#71132);
#13781=VERTEX_POINT('',#71136);
#13782=VERTEX_POINT('',#71140);
#13783=VERTEX_POINT('',#71144);
#13784=VERTEX_POINT('',#71148);
#13785=VERTEX_POINT('',#71152);
#13786=VERTEX_POINT('',#71156);
#13787=VERTEX_POINT('',#71157);
#13788=VERTEX_POINT('',#71159);
#13789=VERTEX_POINT('',#71161);
#13790=VERTEX_POINT('',#71164);
#13791=VERTEX_POINT('',#71166);
#13792=VERTEX_POINT('',#71168);
#13793=VERTEX_POINT('',#71170);
#13794=VERTEX_POINT('',#71172);
#13795=VERTEX_POINT('',#71174);
#13796=VERTEX_POINT('',#71176);
#13797=VERTEX_POINT('',#71178);
#13798=VERTEX_POINT('',#71180);
#13799=VERTEX_POINT('',#71182);
#13800=VERTEX_POINT('',#71193);
#13801=VERTEX_POINT('',#71197);
#13802=VERTEX_POINT('',#71201);
#13803=VERTEX_POINT('',#71205);
#13804=VERTEX_POINT('',#71206);
#13805=VERTEX_POINT('',#71208);
#13806=VERTEX_POINT('',#71210);
#13807=VERTEX_POINT('',#71213);
#13808=VERTEX_POINT('',#71215);
#13809=VERTEX_POINT('',#71217);
#13810=VERTEX_POINT('',#71219);
#13811=VERTEX_POINT('',#71221);
#13812=VERTEX_POINT('',#71223);
#13813=VERTEX_POINT('',#71225);
#13814=VERTEX_POINT('',#71227);
#13815=VERTEX_POINT('',#71229);
#13816=VERTEX_POINT('',#71231);
#13817=VERTEX_POINT('',#71245);
#13818=VERTEX_POINT('',#71249);
#13819=VERTEX_POINT('',#71258);
#13820=VERTEX_POINT('',#71262);
#13821=VERTEX_POINT('',#71268);
#13822=VERTEX_POINT('',#71272);
#13823=VERTEX_POINT('',#71302);
#13824=VERTEX_POINT('',#71303);
#13825=VERTEX_POINT('',#71306);
#13826=VERTEX_POINT('',#71310);
#13827=VERTEX_POINT('',#71312);
#13828=VERTEX_POINT('',#71316);
#13829=VERTEX_POINT('',#71321);
#13830=VERTEX_POINT('',#71325);
#13831=VERTEX_POINT('',#71329);
#13832=VERTEX_POINT('',#71333);
#13833=VERTEX_POINT('',#71341);
#13834=VERTEX_POINT('',#71342);
#13835=VERTEX_POINT('',#71344);
#13836=VERTEX_POINT('',#71346);
#13837=VERTEX_POINT('',#71348);
#13838=VERTEX_POINT('',#71350);
#13839=VERTEX_POINT('',#71352);
#13840=VERTEX_POINT('',#71354);
#13841=VERTEX_POINT('',#71358);
#13842=VERTEX_POINT('',#71363);
#17653=EDGE_CURVE('',#13691,#13691,#2611,.T.);
#17654=EDGE_CURVE('',#13691,#13692,#8644,.T.);
#17655=EDGE_CURVE('',#13692,#13692,#2612,.T.);
#17656=EDGE_CURVE('',#13693,#13694,#8645,.T.);
#17657=EDGE_CURVE('',#13695,#13693,#8646,.T.);
#17658=EDGE_CURVE('',#13696,#13695,#8647,.T.);
#17659=EDGE_CURVE('',#13694,#13696,#8648,.T.);
#17660=EDGE_CURVE('',#13697,#13697,#2613,.T.);
#17661=EDGE_CURVE('',#13698,#13698,#2614,.T.);
#17662=EDGE_CURVE('',#13699,#13699,#2615,.T.);
#17663=EDGE_CURVE('',#13700,#13700,#2616,.T.);
#17664=EDGE_CURVE('',#13701,#13701,#2617,.T.);
#17665=EDGE_CURVE('',#13702,#13702,#2618,.T.);
#17666=EDGE_CURVE('',#13703,#13703,#2619,.T.);
#17667=EDGE_CURVE('',#13704,#13704,#2620,.T.);
#17668=EDGE_CURVE('',#13705,#13705,#2621,.T.);
#17669=EDGE_CURVE('',#13706,#13706,#2622,.T.);
#17670=EDGE_CURVE('',#13692,#13707,#8649,.T.);
#17671=EDGE_CURVE('',#13707,#13707,#2623,.T.);
#17672=EDGE_CURVE('',#13697,#13708,#8650,.T.);
#17673=EDGE_CURVE('',#13708,#13708,#2624,.T.);
#17674=EDGE_CURVE('',#13708,#13709,#8651,.T.);
#17675=EDGE_CURVE('',#13709,#13709,#2625,.T.);
#17676=EDGE_CURVE('',#13706,#13710,#8652,.T.);
#17677=EDGE_CURVE('',#13710,#13710,#2626,.T.);
#17678=EDGE_CURVE('',#13710,#13711,#8653,.T.);
#17679=EDGE_CURVE('',#13711,#13711,#2627,.T.);
#17680=EDGE_CURVE('',#13698,#13712,#8654,.T.);
#17681=EDGE_CURVE('',#13712,#13712,#2628,.T.);
#17682=EDGE_CURVE('',#13712,#13713,#8655,.T.);
#17683=EDGE_CURVE('',#13713,#13713,#2629,.T.);
#17684=EDGE_CURVE('',#13705,#13714,#8656,.T.);
#17685=EDGE_CURVE('',#13714,#13714,#2630,.T.);
#17686=EDGE_CURVE('',#13714,#13715,#8657,.T.);
#17687=EDGE_CURVE('',#13715,#13715,#2631,.T.);
#17688=EDGE_CURVE('',#13699,#13716,#8658,.T.);
#17689=EDGE_CURVE('',#13716,#13716,#2632,.T.);
#17690=EDGE_CURVE('',#13716,#13717,#8659,.T.);
#17691=EDGE_CURVE('',#13717,#13717,#2633,.T.);
#17692=EDGE_CURVE('',#13704,#13718,#8660,.T.);
#17693=EDGE_CURVE('',#13718,#13718,#2634,.T.);
#17694=EDGE_CURVE('',#13718,#13719,#8661,.T.);
#17695=EDGE_CURVE('',#13719,#13719,#2635,.T.);
#17696=EDGE_CURVE('',#13720,#13720,#2636,.T.);
#17697=EDGE_CURVE('',#13720,#13721,#8662,.T.);
#17698=EDGE_CURVE('',#13721,#13721,#2637,.T.);
#17699=EDGE_CURVE('',#13722,#13723,#8663,.T.);
#17700=EDGE_CURVE('',#13724,#13722,#8664,.T.);
#17701=EDGE_CURVE('',#13725,#13724,#8665,.T.);
#17702=EDGE_CURVE('',#13723,#13725,#8666,.T.);
#17703=EDGE_CURVE('',#13726,#13726,#2638,.T.);
#17704=EDGE_CURVE('',#13727,#13727,#2639,.T.);
#17705=EDGE_CURVE('',#13728,#13728,#2640,.T.);
#17706=EDGE_CURVE('',#13729,#13729,#2641,.T.);
#17707=EDGE_CURVE('',#13730,#13730,#2642,.T.);
#17708=EDGE_CURVE('',#13731,#13731,#2643,.T.);
#17709=EDGE_CURVE('',#13732,#13732,#2644,.T.);
#17710=EDGE_CURVE('',#13733,#13733,#2645,.T.);
#17711=EDGE_CURVE('',#13734,#13734,#2646,.T.);
#17712=EDGE_CURVE('',#13735,#13735,#2647,.T.);
#17713=EDGE_CURVE('',#13736,#13736,#2648,.T.);
#17714=EDGE_CURVE('',#13736,#13721,#8667,.T.);
#17715=EDGE_CURVE('',#13726,#13737,#8668,.T.);
#17716=EDGE_CURVE('',#13737,#13737,#2649,.T.);
#17717=EDGE_CURVE('',#13738,#13738,#2650,.T.);
#17718=EDGE_CURVE('',#13738,#13737,#8669,.T.);
#17719=EDGE_CURVE('',#13735,#13739,#8670,.T.);
#17720=EDGE_CURVE('',#13739,#13739,#2651,.T.);
#17721=EDGE_CURVE('',#13740,#13740,#2652,.T.);
#17722=EDGE_CURVE('',#13740,#13739,#8671,.T.);
#17723=EDGE_CURVE('',#13727,#13741,#8672,.T.);
#17724=EDGE_CURVE('',#13741,#13741,#2653,.T.);
#17725=EDGE_CURVE('',#13742,#13742,#2654,.T.);
#17726=EDGE_CURVE('',#13742,#13741,#8673,.T.);
#17727=EDGE_CURVE('',#13734,#13743,#8674,.T.);
#17728=EDGE_CURVE('',#13743,#13743,#2655,.T.);
#17729=EDGE_CURVE('',#13744,#13744,#2656,.T.);
#17730=EDGE_CURVE('',#13744,#13743,#8675,.T.);
#17731=EDGE_CURVE('',#13745,#13722,#8676,.T.);
#17732=EDGE_CURVE('',#13723,#13746,#8677,.T.);
#17733=EDGE_CURVE('',#13746,#13745,#8678,.T.);
#17734=EDGE_CURVE('',#13747,#13748,#8679,.T.);
#17735=EDGE_CURVE('',#13748,#13722,#2657,.T.);
#17736=EDGE_CURVE('',#13745,#13747,#2658,.T.);
#17737=EDGE_CURVE('',#13749,#13750,#8680,.T.);
#17738=EDGE_CURVE('',#13750,#13748,#8681,.T.);
#17739=EDGE_CURVE('',#13747,#13749,#8682,.T.);
#17740=EDGE_CURVE('',#13751,#13694,#8683,.T.);
#17741=EDGE_CURVE('',#13694,#13750,#2659,.T.);
#17742=EDGE_CURVE('',#13749,#13751,#2660,.T.);
#17743=EDGE_CURVE('',#13752,#13693,#8684,.T.);
#17744=EDGE_CURVE('',#13751,#13752,#8685,.T.);
#17745=EDGE_CURVE('',#13753,#13754,#8686,.T.);
#17746=EDGE_CURVE('',#13754,#13693,#2661,.T.);
#17747=EDGE_CURVE('',#13752,#13753,#2662,.T.);
#17748=EDGE_CURVE('',#13755,#13756,#8687,.T.);
#17749=EDGE_CURVE('',#13756,#13754,#8688,.T.);
#17750=EDGE_CURVE('',#13753,#13755,#8689,.T.);
#17751=EDGE_CURVE('',#13723,#13756,#2663,.T.);
#17752=EDGE_CURVE('',#13755,#13746,#2664,.T.);
#17753=EDGE_CURVE('',#13754,#13757,#8690,.T.);
#17754=EDGE_CURVE('',#13695,#13757,#2665,.T.);
#17755=EDGE_CURVE('',#13758,#13756,#8691,.T.);
#17756=EDGE_CURVE('',#13757,#13758,#8692,.T.);
#17757=EDGE_CURVE('',#13758,#13725,#2666,.T.);
#17758=EDGE_CURVE('',#13759,#13760,#8693,.T.);
#17759=EDGE_CURVE('',#13761,#13759,#2667,.T.);
#17760=EDGE_CURVE('',#13762,#13761,#8694,.T.);
#17761=EDGE_CURVE('',#13763,#13762,#2668,.T.);
#17762=EDGE_CURVE('',#13764,#13763,#8695,.T.);
#17763=EDGE_CURVE('',#13765,#13764,#2669,.T.);
#17764=EDGE_CURVE('',#13766,#13765,#8696,.T.);
#17765=EDGE_CURVE('',#13760,#13766,#2670,.T.);
#17766=EDGE_CURVE('',#13733,#13767,#8697,.T.);
#17767=EDGE_CURVE('',#13767,#13767,#2671,.T.);
#17768=EDGE_CURVE('',#13768,#13768,#2672,.T.);
#17769=EDGE_CURVE('',#13768,#13767,#8698,.T.);
#17770=EDGE_CURVE('',#13728,#13769,#8699,.T.);
#17771=EDGE_CURVE('',#13769,#13769,#2673,.T.);
#17772=EDGE_CURVE('',#13770,#13770,#2674,.T.);
#17773=EDGE_CURVE('',#13770,#13769,#8700,.T.);
#17774=EDGE_CURVE('',#13732,#13771,#8701,.T.);
#17775=EDGE_CURVE('',#13771,#13771,#2675,.T.);
#17776=EDGE_CURVE('',#13772,#13772,#2676,.T.);
#17777=EDGE_CURVE('',#13772,#13771,#8702,.T.);
#17778=EDGE_CURVE('',#13700,#13773,#8703,.T.);
#17779=EDGE_CURVE('',#13773,#13773,#2677,.T.);
#17780=EDGE_CURVE('',#13773,#13774,#8704,.T.);
#17781=EDGE_CURVE('',#13774,#13774,#2678,.T.);
#17782=EDGE_CURVE('',#13729,#13775,#8705,.T.);
#17783=EDGE_CURVE('',#13775,#13775,#2679,.T.);
#17784=EDGE_CURVE('',#13776,#13776,#2680,.T.);
#17785=EDGE_CURVE('',#13776,#13775,#8706,.T.);
#17786=EDGE_CURVE('',#13703,#13777,#8707,.T.);
#17787=EDGE_CURVE('',#13777,#13777,#2681,.T.);
#17788=EDGE_CURVE('',#13777,#13778,#8708,.T.);
#17789=EDGE_CURVE('',#13778,#13778,#2682,.T.);
#17790=EDGE_CURVE('',#13731,#13779,#8709,.T.);
#17791=EDGE_CURVE('',#13779,#13779,#2683,.T.);
#17792=EDGE_CURVE('',#13780,#13780,#2684,.T.);
#17793=EDGE_CURVE('',#13780,#13779,#8710,.T.);
#17794=EDGE_CURVE('',#13701,#13781,#8711,.T.);
#17795=EDGE_CURVE('',#13781,#13781,#2685,.T.);
#17796=EDGE_CURVE('',#13781,#13782,#8712,.T.);
#17797=EDGE_CURVE('',#13782,#13782,#2686,.T.);
#17798=EDGE_CURVE('',#13730,#13783,#8713,.T.);
#17799=EDGE_CURVE('',#13783,#13783,#2687,.T.);
#17800=EDGE_CURVE('',#13784,#13784,#2688,.T.);
#17801=EDGE_CURVE('',#13784,#13783,#8714,.T.);
#17802=EDGE_CURVE('',#13785,#13785,#2689,.T.);
#17803=EDGE_CURVE('',#13785,#13736,#8715,.T.);
#17804=EDGE_CURVE('',#13786,#13787,#8716,.T.);
#17805=EDGE_CURVE('',#13788,#13786,#8717,.T.);
#17806=EDGE_CURVE('',#13789,#13788,#8718,.T.);
#17807=EDGE_CURVE('',#13787,#13789,#8719,.T.);
#17808=EDGE_CURVE('',#13790,#13790,#2690,.T.);
#17809=EDGE_CURVE('',#13791,#13791,#2691,.T.);
#17810=EDGE_CURVE('',#13792,#13792,#2692,.T.);
#17811=EDGE_CURVE('',#13793,#13793,#2693,.T.);
#17812=EDGE_CURVE('',#13794,#13794,#2694,.T.);
#17813=EDGE_CURVE('',#13795,#13795,#2695,.T.);
#17814=EDGE_CURVE('',#13796,#13796,#2696,.T.);
#17815=EDGE_CURVE('',#13797,#13797,#2697,.T.);
#17816=EDGE_CURVE('',#13798,#13798,#2698,.T.);
#17817=EDGE_CURVE('',#13799,#13799,#2699,.T.);
#17818=EDGE_CURVE('',#13790,#13738,#8720,.T.);
#17819=EDGE_CURVE('',#13799,#13740,#8721,.T.);
#17820=EDGE_CURVE('',#13791,#13742,#8722,.T.);
#17821=EDGE_CURVE('',#13798,#13744,#8723,.T.);
#17822=EDGE_CURVE('',#13702,#13800,#8724,.T.);
#17823=EDGE_CURVE('',#13800,#13800,#2700,.T.);
#17824=EDGE_CURVE('',#13800,#13801,#8725,.T.);
#17825=EDGE_CURVE('',#13801,#13801,#2701,.T.);
#17826=EDGE_CURVE('',#13802,#13802,#2702,.T.);
#17827=EDGE_CURVE('',#13802,#13707,#8726,.T.);
#17828=EDGE_CURVE('',#13803,#13804,#8727,.T.);
#17829=EDGE_CURVE('',#13805,#13803,#8728,.T.);
#17830=EDGE_CURVE('',#13806,#13805,#8729,.T.);
#17831=EDGE_CURVE('',#13804,#13806,#8730,.T.);
#17832=EDGE_CURVE('',#13807,#13807,#2703,.T.);
#17833=EDGE_CURVE('',#13808,#13808,#2704,.T.);
#17834=EDGE_CURVE('',#13809,#13809,#2705,.T.);
#17835=EDGE_CURVE('',#13810,#13810,#2706,.T.);
#17836=EDGE_CURVE('',#13811,#13811,#2707,.T.);
#17837=EDGE_CURVE('',#13812,#13812,#2708,.T.);
#17838=EDGE_CURVE('',#13813,#13813,#2709,.T.);
#17839=EDGE_CURVE('',#13814,#13814,#2710,.T.);
#17840=EDGE_CURVE('',#13815,#13815,#2711,.T.);
#17841=EDGE_CURVE('',#13816,#13816,#2712,.T.);
#17842=EDGE_CURVE('',#13807,#13709,#8731,.T.);
#17843=EDGE_CURVE('',#13816,#13711,#8732,.T.);
#17844=EDGE_CURVE('',#13808,#13713,#8733,.T.);
#17845=EDGE_CURVE('',#13815,#13715,#8734,.T.);
#17846=EDGE_CURVE('',#13760,#13803,#8735,.T.);
#17847=EDGE_CURVE('',#13804,#13759,#8736,.T.);
#17848=EDGE_CURVE('',#13766,#13817,#8737,.T.);
#17849=EDGE_CURVE('',#13817,#13803,#2713,.T.);
#17850=EDGE_CURVE('',#13765,#13818,#8738,.T.);
#17851=EDGE_CURVE('',#13818,#13817,#8739,.T.);
#17852=EDGE_CURVE('',#13764,#13787,#8740,.T.);
#17853=EDGE_CURVE('',#13787,#13818,#2714,.T.);
#17854=EDGE_CURVE('',#13763,#13786,#8741,.T.);
#17855=EDGE_CURVE('',#13762,#13819,#8742,.T.);
#17856=EDGE_CURVE('',#13819,#13786,#2715,.T.);
#17857=EDGE_CURVE('',#13761,#13820,#8743,.T.);
#17858=EDGE_CURVE('',#13820,#13819,#8744,.T.);
#17859=EDGE_CURVE('',#13804,#13820,#2716,.T.);
#17860=EDGE_CURVE('',#13819,#13821,#8745,.T.);
#17861=EDGE_CURVE('',#13788,#13821,#2717,.T.);
#17862=EDGE_CURVE('',#13822,#13820,#8746,.T.);
#17863=EDGE_CURVE('',#13821,#13822,#8747,.T.);
#17864=EDGE_CURVE('',#13822,#13806,#2718,.T.);
#17865=EDGE_CURVE('',#13814,#13801,#8748,.T.);
#17866=EDGE_CURVE('',#13792,#13784,#8749,.T.);
#17867=EDGE_CURVE('',#13809,#13782,#8750,.T.);
#17868=EDGE_CURVE('',#13797,#13780,#8751,.T.);
#17869=EDGE_CURVE('',#13813,#13778,#8752,.T.);
#17870=EDGE_CURVE('',#13793,#13776,#8753,.T.);
#17871=EDGE_CURVE('',#13810,#13774,#8754,.T.);
#17872=EDGE_CURVE('',#13796,#13772,#8755,.T.);
#17873=EDGE_CURVE('',#13812,#13717,#8756,.T.);
#17874=EDGE_CURVE('',#13794,#13768,#8757,.T.);
#17875=EDGE_CURVE('',#13811,#13719,#8758,.T.);
#17876=EDGE_CURVE('',#13795,#13770,#8759,.T.);
#17877=EDGE_CURVE('',#13823,#13824,#8760,.T.);
#17878=EDGE_CURVE('',#13824,#13789,#2719,.T.);
#17879=EDGE_CURVE('',#13789,#13825,#8761,.T.);
#17880=EDGE_CURVE('',#13825,#13823,#2720,.T.);
#17881=EDGE_CURVE('',#13823,#13826,#8762,.T.);
#17882=EDGE_CURVE('',#13826,#13827,#8763,.T.);
#17883=EDGE_CURVE('',#13827,#13824,#8764,.T.);
#17884=EDGE_CURVE('',#13828,#13805,#8765,.T.);
#17885=EDGE_CURVE('',#13805,#13827,#2721,.T.);
#17886=EDGE_CURVE('',#13826,#13828,#2722,.T.);
#17887=EDGE_CURVE('',#13828,#13829,#8766,.T.);
#17888=EDGE_CURVE('',#13829,#13806,#8767,.T.);
#17889=EDGE_CURVE('',#13830,#13822,#8768,.T.);
#17890=EDGE_CURVE('',#13829,#13830,#2723,.T.);
#17891=EDGE_CURVE('',#13830,#13831,#8769,.T.);
#17892=EDGE_CURVE('',#13831,#13821,#8770,.T.);
#17893=EDGE_CURVE('',#13832,#13788,#8771,.T.);
#17894=EDGE_CURVE('',#13831,#13832,#2724,.T.);
#17895=EDGE_CURVE('',#13832,#13825,#8772,.T.);
#17896=EDGE_CURVE('',#13824,#13818,#8773,.T.);
#17897=EDGE_CURVE('',#13833,#13834,#2725,.T.);
#17898=EDGE_CURVE('',#13835,#13833,#8774,.T.);
#17899=EDGE_CURVE('',#13836,#13835,#2726,.T.);
#17900=EDGE_CURVE('',#13837,#13836,#8775,.T.);
#17901=EDGE_CURVE('',#13838,#13837,#2727,.T.);
#17902=EDGE_CURVE('',#13839,#13838,#8776,.T.);
#17903=EDGE_CURVE('',#13840,#13839,#2728,.T.);
#17904=EDGE_CURVE('',#13834,#13840,#8777,.T.);
#17905=EDGE_CURVE('',#13834,#13841,#8778,.T.);
#17906=EDGE_CURVE('',#13841,#13696,#2729,.T.);
#17907=EDGE_CURVE('',#13696,#13833,#8779,.T.);
#17908=EDGE_CURVE('',#13840,#13842,#8780,.T.);
#17909=EDGE_CURVE('',#13842,#13841,#8781,.T.);
#17910=EDGE_CURVE('',#13839,#13724,#8782,.T.);
#17911=EDGE_CURVE('',#13724,#13842,#2730,.T.);
#17912=EDGE_CURVE('',#13838,#13725,#8783,.T.);
#17913=EDGE_CURVE('',#13837,#13758,#8784,.T.);
#17914=EDGE_CURVE('',#13836,#13757,#8785,.T.);
#17915=EDGE_CURVE('',#13835,#13695,#8786,.T.);
#17916=EDGE_CURVE('',#13841,#13750,#8787,.T.);
#17917=EDGE_CURVE('',#13748,#13842,#8788,.T.);
#17918=EDGE_CURVE('',#13817,#13827,#8789,.T.);
#25539=ORIENTED_EDGE('',*,*,#17653,.T.);
#25540=ORIENTED_EDGE('',*,*,#17654,.T.);
#25541=ORIENTED_EDGE('',*,*,#17655,.T.);
#25542=ORIENTED_EDGE('',*,*,#17654,.F.);
#25543=ORIENTED_EDGE('',*,*,#17656,.F.);
#25544=ORIENTED_EDGE('',*,*,#17657,.F.);
#25545=ORIENTED_EDGE('',*,*,#17658,.F.);
#25546=ORIENTED_EDGE('',*,*,#17659,.F.);
#25547=ORIENTED_EDGE('',*,*,#17660,.F.);
#25548=ORIENTED_EDGE('',*,*,#17661,.F.);
#25549=ORIENTED_EDGE('',*,*,#17662,.F.);
#25550=ORIENTED_EDGE('',*,*,#17663,.F.);
#25551=ORIENTED_EDGE('',*,*,#17664,.F.);
#25552=ORIENTED_EDGE('',*,*,#17665,.F.);
#25553=ORIENTED_EDGE('',*,*,#17666,.F.);
#25554=ORIENTED_EDGE('',*,*,#17667,.F.);
#25555=ORIENTED_EDGE('',*,*,#17668,.F.);
#25556=ORIENTED_EDGE('',*,*,#17669,.F.);
#25557=ORIENTED_EDGE('',*,*,#17653,.F.);
#25558=ORIENTED_EDGE('',*,*,#17655,.F.);
#25559=ORIENTED_EDGE('',*,*,#17670,.T.);
#25560=ORIENTED_EDGE('',*,*,#17671,.F.);
#25561=ORIENTED_EDGE('',*,*,#17670,.F.);
#25562=ORIENTED_EDGE('',*,*,#17660,.T.);
#25563=ORIENTED_EDGE('',*,*,#17672,.T.);
#25564=ORIENTED_EDGE('',*,*,#17673,.T.);
#25565=ORIENTED_EDGE('',*,*,#17672,.F.);
#25566=ORIENTED_EDGE('',*,*,#17673,.F.);
#25567=ORIENTED_EDGE('',*,*,#17674,.T.);
#25568=ORIENTED_EDGE('',*,*,#17675,.F.);
#25569=ORIENTED_EDGE('',*,*,#17674,.F.);
#25570=ORIENTED_EDGE('',*,*,#17669,.T.);
#25571=ORIENTED_EDGE('',*,*,#17676,.T.);
#25572=ORIENTED_EDGE('',*,*,#17677,.T.);
#25573=ORIENTED_EDGE('',*,*,#17676,.F.);
#25574=ORIENTED_EDGE('',*,*,#17677,.F.);
#25575=ORIENTED_EDGE('',*,*,#17678,.T.);
#25576=ORIENTED_EDGE('',*,*,#17679,.F.);
#25577=ORIENTED_EDGE('',*,*,#17678,.F.);
#25578=ORIENTED_EDGE('',*,*,#17661,.T.);
#25579=ORIENTED_EDGE('',*,*,#17680,.T.);
#25580=ORIENTED_EDGE('',*,*,#17681,.T.);
#25581=ORIENTED_EDGE('',*,*,#17680,.F.);
#25582=ORIENTED_EDGE('',*,*,#17681,.F.);
#25583=ORIENTED_EDGE('',*,*,#17682,.T.);
#25584=ORIENTED_EDGE('',*,*,#17683,.F.);
#25585=ORIENTED_EDGE('',*,*,#17682,.F.);
#25586=ORIENTED_EDGE('',*,*,#17668,.T.);
#25587=ORIENTED_EDGE('',*,*,#17684,.T.);
#25588=ORIENTED_EDGE('',*,*,#17685,.T.);
#25589=ORIENTED_EDGE('',*,*,#17684,.F.);
#25590=ORIENTED_EDGE('',*,*,#17685,.F.);
#25591=ORIENTED_EDGE('',*,*,#17686,.T.);
#25592=ORIENTED_EDGE('',*,*,#17687,.F.);
#25593=ORIENTED_EDGE('',*,*,#17686,.F.);
#25594=ORIENTED_EDGE('',*,*,#17662,.T.);
#25595=ORIENTED_EDGE('',*,*,#17688,.T.);
#25596=ORIENTED_EDGE('',*,*,#17689,.T.);
#25597=ORIENTED_EDGE('',*,*,#17688,.F.);
#25598=ORIENTED_EDGE('',*,*,#17689,.F.);
#25599=ORIENTED_EDGE('',*,*,#17690,.T.);
#25600=ORIENTED_EDGE('',*,*,#17691,.F.);
#25601=ORIENTED_EDGE('',*,*,#17690,.F.);
#25602=ORIENTED_EDGE('',*,*,#17667,.T.);
#25603=ORIENTED_EDGE('',*,*,#17692,.T.);
#25604=ORIENTED_EDGE('',*,*,#17693,.T.);
#25605=ORIENTED_EDGE('',*,*,#17692,.F.);
#25606=ORIENTED_EDGE('',*,*,#17693,.F.);
#25607=ORIENTED_EDGE('',*,*,#17694,.T.);
#25608=ORIENTED_EDGE('',*,*,#17695,.F.);
#25609=ORIENTED_EDGE('',*,*,#17694,.F.);
#25610=ORIENTED_EDGE('',*,*,#17696,.T.);
#25611=ORIENTED_EDGE('',*,*,#17697,.T.);
#25612=ORIENTED_EDGE('',*,*,#17698,.T.);
#25613=ORIENTED_EDGE('',*,*,#17697,.F.);
#25614=ORIENTED_EDGE('',*,*,#17699,.F.);
#25615=ORIENTED_EDGE('',*,*,#17700,.F.);
#25616=ORIENTED_EDGE('',*,*,#17701,.F.);
#25617=ORIENTED_EDGE('',*,*,#17702,.F.);
#25618=ORIENTED_EDGE('',*,*,#17703,.F.);
#25619=ORIENTED_EDGE('',*,*,#17704,.F.);
#25620=ORIENTED_EDGE('',*,*,#17705,.F.);
#25621=ORIENTED_EDGE('',*,*,#17706,.F.);
#25622=ORIENTED_EDGE('',*,*,#17707,.F.);
#25623=ORIENTED_EDGE('',*,*,#17708,.F.);
#25624=ORIENTED_EDGE('',*,*,#17709,.F.);
#25625=ORIENTED_EDGE('',*,*,#17710,.F.);
#25626=ORIENTED_EDGE('',*,*,#17711,.F.);
#25627=ORIENTED_EDGE('',*,*,#17712,.F.);
#25628=ORIENTED_EDGE('',*,*,#17696,.F.);
#25629=ORIENTED_EDGE('',*,*,#17713,.F.);
#25630=ORIENTED_EDGE('',*,*,#17714,.T.);
#25631=ORIENTED_EDGE('',*,*,#17698,.F.);
#25632=ORIENTED_EDGE('',*,*,#17714,.F.);
#25633=ORIENTED_EDGE('',*,*,#17703,.T.);
#25634=ORIENTED_EDGE('',*,*,#17715,.T.);
#25635=ORIENTED_EDGE('',*,*,#17716,.T.);
#25636=ORIENTED_EDGE('',*,*,#17715,.F.);
#25637=ORIENTED_EDGE('',*,*,#17717,.F.);
#25638=ORIENTED_EDGE('',*,*,#17718,.T.);
#25639=ORIENTED_EDGE('',*,*,#17716,.F.);
#25640=ORIENTED_EDGE('',*,*,#17718,.F.);
#25641=ORIENTED_EDGE('',*,*,#17712,.T.);
#25642=ORIENTED_EDGE('',*,*,#17719,.T.);
#25643=ORIENTED_EDGE('',*,*,#17720,.T.);
#25644=ORIENTED_EDGE('',*,*,#17719,.F.);
#25645=ORIENTED_EDGE('',*,*,#17721,.F.);
#25646=ORIENTED_EDGE('',*,*,#17722,.T.);
#25647=ORIENTED_EDGE('',*,*,#17720,.F.);
#25648=ORIENTED_EDGE('',*,*,#17722,.F.);
#25649=ORIENTED_EDGE('',*,*,#17704,.T.);
#25650=ORIENTED_EDGE('',*,*,#17723,.T.);
#25651=ORIENTED_EDGE('',*,*,#17724,.T.);
#25652=ORIENTED_EDGE('',*,*,#17723,.F.);
#25653=ORIENTED_EDGE('',*,*,#17725,.F.);
#25654=ORIENTED_EDGE('',*,*,#17726,.T.);
#25655=ORIENTED_EDGE('',*,*,#17724,.F.);
#25656=ORIENTED_EDGE('',*,*,#17726,.F.);
#25657=ORIENTED_EDGE('',*,*,#17711,.T.);
#25658=ORIENTED_EDGE('',*,*,#17727,.T.);
#25659=ORIENTED_EDGE('',*,*,#17728,.T.);
#25660=ORIENTED_EDGE('',*,*,#17727,.F.);
#25661=ORIENTED_EDGE('',*,*,#17729,.F.);
#25662=ORIENTED_EDGE('',*,*,#17730,.T.);
#25663=ORIENTED_EDGE('',*,*,#17728,.F.);
#25664=ORIENTED_EDGE('',*,*,#17730,.F.);
#25665=ORIENTED_EDGE('',*,*,#17731,.T.);
#25666=ORIENTED_EDGE('',*,*,#17699,.T.);
#25667=ORIENTED_EDGE('',*,*,#17732,.T.);
#25668=ORIENTED_EDGE('',*,*,#17733,.T.);
#25669=ORIENTED_EDGE('',*,*,#17734,.T.);
#25670=ORIENTED_EDGE('',*,*,#17735,.T.);
#25671=ORIENTED_EDGE('',*,*,#17731,.F.);
#25672=ORIENTED_EDGE('',*,*,#17736,.T.);
#25673=ORIENTED_EDGE('',*,*,#17737,.T.);
#25674=ORIENTED_EDGE('',*,*,#17738,.T.);
#25675=ORIENTED_EDGE('',*,*,#17734,.F.);
#25676=ORIENTED_EDGE('',*,*,#17739,.T.);
#25677=ORIENTED_EDGE('',*,*,#17740,.T.);
#25678=ORIENTED_EDGE('',*,*,#17741,.T.);
#25679=ORIENTED_EDGE('',*,*,#17737,.F.);
#25680=ORIENTED_EDGE('',*,*,#17742,.T.);
#25681=ORIENTED_EDGE('',*,*,#17743,.T.);
#25682=ORIENTED_EDGE('',*,*,#17656,.T.);
#25683=ORIENTED_EDGE('',*,*,#17740,.F.);
#25684=ORIENTED_EDGE('',*,*,#17744,.T.);
#25685=ORIENTED_EDGE('',*,*,#17745,.T.);
#25686=ORIENTED_EDGE('',*,*,#17746,.T.);
#25687=ORIENTED_EDGE('',*,*,#17743,.F.);
#25688=ORIENTED_EDGE('',*,*,#17747,.T.);
#25689=ORIENTED_EDGE('',*,*,#17748,.T.);
#25690=ORIENTED_EDGE('',*,*,#17749,.T.);
#25691=ORIENTED_EDGE('',*,*,#17745,.F.);
#25692=ORIENTED_EDGE('',*,*,#17750,.T.);
#25693=ORIENTED_EDGE('',*,*,#17732,.F.);
#25694=ORIENTED_EDGE('',*,*,#17751,.T.);
#25695=ORIENTED_EDGE('',*,*,#17748,.F.);
#25696=ORIENTED_EDGE('',*,*,#17752,.T.);
#25697=ORIENTED_EDGE('',*,*,#17746,.F.);
#25698=ORIENTED_EDGE('',*,*,#17753,.T.);
#25699=ORIENTED_EDGE('',*,*,#17754,.F.);
#25700=ORIENTED_EDGE('',*,*,#17657,.T.);
#25701=ORIENTED_EDGE('',*,*,#17749,.F.);
#25702=ORIENTED_EDGE('',*,*,#17755,.F.);
#25703=ORIENTED_EDGE('',*,*,#17756,.F.);
#25704=ORIENTED_EDGE('',*,*,#17753,.F.);
#25705=ORIENTED_EDGE('',*,*,#17751,.F.);
#25706=ORIENTED_EDGE('',*,*,#17702,.T.);
#25707=ORIENTED_EDGE('',*,*,#17757,.F.);
#25708=ORIENTED_EDGE('',*,*,#17755,.T.);
#25709=ORIENTED_EDGE('',*,*,#17758,.F.);
#25710=ORIENTED_EDGE('',*,*,#17759,.F.);
#25711=ORIENTED_EDGE('',*,*,#17760,.F.);
#25712=ORIENTED_EDGE('',*,*,#17761,.F.);
#25713=ORIENTED_EDGE('',*,*,#17762,.F.);
#25714=ORIENTED_EDGE('',*,*,#17763,.F.);
#25715=ORIENTED_EDGE('',*,*,#17764,.F.);
#25716=ORIENTED_EDGE('',*,*,#17765,.F.);
#25717=ORIENTED_EDGE('',*,*,#17733,.F.);
#25718=ORIENTED_EDGE('',*,*,#17752,.F.);
#25719=ORIENTED_EDGE('',*,*,#17750,.F.);
#25720=ORIENTED_EDGE('',*,*,#17747,.F.);
#25721=ORIENTED_EDGE('',*,*,#17744,.F.);
#25722=ORIENTED_EDGE('',*,*,#17742,.F.);
#25723=ORIENTED_EDGE('',*,*,#17739,.F.);
#25724=ORIENTED_EDGE('',*,*,#17736,.F.);
#25725=ORIENTED_EDGE('',*,*,#17710,.T.);
#25726=ORIENTED_EDGE('',*,*,#17766,.T.);
#25727=ORIENTED_EDGE('',*,*,#17767,.T.);
#25728=ORIENTED_EDGE('',*,*,#17766,.F.);
#25729=ORIENTED_EDGE('',*,*,#17768,.F.);
#25730=ORIENTED_EDGE('',*,*,#17769,.T.);
#25731=ORIENTED_EDGE('',*,*,#17767,.F.);
#25732=ORIENTED_EDGE('',*,*,#17769,.F.);
#25733=ORIENTED_EDGE('',*,*,#17705,.T.);
#25734=ORIENTED_EDGE('',*,*,#17770,.T.);
#25735=ORIENTED_EDGE('',*,*,#17771,.T.);
#25736=ORIENTED_EDGE('',*,*,#17770,.F.);
#25737=ORIENTED_EDGE('',*,*,#17772,.F.);
#25738=ORIENTED_EDGE('',*,*,#17773,.T.);
#25739=ORIENTED_EDGE('',*,*,#17771,.F.);
#25740=ORIENTED_EDGE('',*,*,#17773,.F.);
#25741=ORIENTED_EDGE('',*,*,#17709,.T.);
#25742=ORIENTED_EDGE('',*,*,#17774,.T.);
#25743=ORIENTED_EDGE('',*,*,#17775,.T.);
#25744=ORIENTED_EDGE('',*,*,#17774,.F.);
#25745=ORIENTED_EDGE('',*,*,#17776,.F.);
#25746=ORIENTED_EDGE('',*,*,#17777,.T.);
#25747=ORIENTED_EDGE('',*,*,#17775,.F.);
#25748=ORIENTED_EDGE('',*,*,#17777,.F.);
#25749=ORIENTED_EDGE('',*,*,#17663,.T.);
#25750=ORIENTED_EDGE('',*,*,#17778,.T.);
#25751=ORIENTED_EDGE('',*,*,#17779,.T.);
#25752=ORIENTED_EDGE('',*,*,#17778,.F.);
#25753=ORIENTED_EDGE('',*,*,#17779,.F.);
#25754=ORIENTED_EDGE('',*,*,#17780,.T.);
#25755=ORIENTED_EDGE('',*,*,#17781,.F.);
#25756=ORIENTED_EDGE('',*,*,#17780,.F.);
#25757=ORIENTED_EDGE('',*,*,#17706,.T.);
#25758=ORIENTED_EDGE('',*,*,#17782,.T.);
#25759=ORIENTED_EDGE('',*,*,#17783,.T.);
#25760=ORIENTED_EDGE('',*,*,#17782,.F.);
#25761=ORIENTED_EDGE('',*,*,#17784,.F.);
#25762=ORIENTED_EDGE('',*,*,#17785,.T.);
#25763=ORIENTED_EDGE('',*,*,#17783,.F.);
#25764=ORIENTED_EDGE('',*,*,#17785,.F.);
#25765=ORIENTED_EDGE('',*,*,#17666,.T.);
#25766=ORIENTED_EDGE('',*,*,#17786,.T.);
#25767=ORIENTED_EDGE('',*,*,#17787,.T.);
#25768=ORIENTED_EDGE('',*,*,#17786,.F.);
#25769=ORIENTED_EDGE('',*,*,#17787,.F.);
#25770=ORIENTED_EDGE('',*,*,#17788,.T.);
#25771=ORIENTED_EDGE('',*,*,#17789,.F.);
#25772=ORIENTED_EDGE('',*,*,#17788,.F.);
#25773=ORIENTED_EDGE('',*,*,#17708,.T.);
#25774=ORIENTED_EDGE('',*,*,#17790,.T.);
#25775=ORIENTED_EDGE('',*,*,#17791,.T.);
#25776=ORIENTED_EDGE('',*,*,#17790,.F.);
#25777=ORIENTED_EDGE('',*,*,#17792,.F.);
#25778=ORIENTED_EDGE('',*,*,#17793,.T.);
#25779=ORIENTED_EDGE('',*,*,#17791,.F.);
#25780=ORIENTED_EDGE('',*,*,#17793,.F.);
#25781=ORIENTED_EDGE('',*,*,#17664,.T.);
#25782=ORIENTED_EDGE('',*,*,#17794,.T.);
#25783=ORIENTED_EDGE('',*,*,#17795,.T.);
#25784=ORIENTED_EDGE('',*,*,#17794,.F.);
#25785=ORIENTED_EDGE('',*,*,#17795,.F.);
#25786=ORIENTED_EDGE('',*,*,#17796,.T.);
#25787=ORIENTED_EDGE('',*,*,#17797,.F.);
#25788=ORIENTED_EDGE('',*,*,#17796,.F.);
#25789=ORIENTED_EDGE('',*,*,#17707,.T.);
#25790=ORIENTED_EDGE('',*,*,#17798,.T.);
#25791=ORIENTED_EDGE('',*,*,#17799,.T.);
#25792=ORIENTED_EDGE('',*,*,#17798,.F.);
#25793=ORIENTED_EDGE('',*,*,#17800,.F.);
#25794=ORIENTED_EDGE('',*,*,#17801,.T.);
#25795=ORIENTED_EDGE('',*,*,#17799,.F.);
#25796=ORIENTED_EDGE('',*,*,#17801,.F.);
#25797=ORIENTED_EDGE('',*,*,#17802,.T.);
#25798=ORIENTED_EDGE('',*,*,#17803,.T.);
#25799=ORIENTED_EDGE('',*,*,#17713,.T.);
#25800=ORIENTED_EDGE('',*,*,#17803,.F.);
#25801=ORIENTED_EDGE('',*,*,#17804,.F.);
#25802=ORIENTED_EDGE('',*,*,#17805,.F.);
#25803=ORIENTED_EDGE('',*,*,#17806,.F.);
#25804=ORIENTED_EDGE('',*,*,#17807,.F.);
#25805=ORIENTED_EDGE('',*,*,#17808,.F.);
#25806=ORIENTED_EDGE('',*,*,#17809,.F.);
#25807=ORIENTED_EDGE('',*,*,#17810,.F.);
#25808=ORIENTED_EDGE('',*,*,#17811,.F.);
#25809=ORIENTED_EDGE('',*,*,#17812,.F.);
#25810=ORIENTED_EDGE('',*,*,#17813,.F.);
#25811=ORIENTED_EDGE('',*,*,#17814,.F.);
#25812=ORIENTED_EDGE('',*,*,#17815,.F.);
#25813=ORIENTED_EDGE('',*,*,#17816,.F.);
#25814=ORIENTED_EDGE('',*,*,#17817,.F.);
#25815=ORIENTED_EDGE('',*,*,#17802,.F.);
#25816=ORIENTED_EDGE('',*,*,#17808,.T.);
#25817=ORIENTED_EDGE('',*,*,#17818,.T.);
#25818=ORIENTED_EDGE('',*,*,#17717,.T.);
#25819=ORIENTED_EDGE('',*,*,#17818,.F.);
#25820=ORIENTED_EDGE('',*,*,#17817,.T.);
#25821=ORIENTED_EDGE('',*,*,#17819,.T.);
#25822=ORIENTED_EDGE('',*,*,#17721,.T.);
#25823=ORIENTED_EDGE('',*,*,#17819,.F.);
#25824=ORIENTED_EDGE('',*,*,#17809,.T.);
#25825=ORIENTED_EDGE('',*,*,#17820,.T.);
#25826=ORIENTED_EDGE('',*,*,#17725,.T.);
#25827=ORIENTED_EDGE('',*,*,#17820,.F.);
#25828=ORIENTED_EDGE('',*,*,#17816,.T.);
#25829=ORIENTED_EDGE('',*,*,#17821,.T.);
#25830=ORIENTED_EDGE('',*,*,#17729,.T.);
#25831=ORIENTED_EDGE('',*,*,#17821,.F.);
#25832=ORIENTED_EDGE('',*,*,#17665,.T.);
#25833=ORIENTED_EDGE('',*,*,#17822,.T.);
#25834=ORIENTED_EDGE('',*,*,#17823,.T.);
#25835=ORIENTED_EDGE('',*,*,#17822,.F.);
#25836=ORIENTED_EDGE('',*,*,#17823,.F.);
#25837=ORIENTED_EDGE('',*,*,#17824,.T.);
#25838=ORIENTED_EDGE('',*,*,#17825,.F.);
#25839=ORIENTED_EDGE('',*,*,#17824,.F.);
#25840=ORIENTED_EDGE('',*,*,#17826,.T.);
#25841=ORIENTED_EDGE('',*,*,#17827,.T.);
#25842=ORIENTED_EDGE('',*,*,#17671,.T.);
#25843=ORIENTED_EDGE('',*,*,#17827,.F.);
#25844=ORIENTED_EDGE('',*,*,#17828,.F.);
#25845=ORIENTED_EDGE('',*,*,#17829,.F.);
#25846=ORIENTED_EDGE('',*,*,#17830,.F.);
#25847=ORIENTED_EDGE('',*,*,#17831,.F.);
#25848=ORIENTED_EDGE('',*,*,#17832,.F.);
#25849=ORIENTED_EDGE('',*,*,#17833,.F.);
#25850=ORIENTED_EDGE('',*,*,#17834,.F.);
#25851=ORIENTED_EDGE('',*,*,#17835,.F.);
#25852=ORIENTED_EDGE('',*,*,#17836,.F.);
#25853=ORIENTED_EDGE('',*,*,#17837,.F.);
#25854=ORIENTED_EDGE('',*,*,#17838,.F.);
#25855=ORIENTED_EDGE('',*,*,#17839,.F.);
#25856=ORIENTED_EDGE('',*,*,#17840,.F.);
#25857=ORIENTED_EDGE('',*,*,#17841,.F.);
#25858=ORIENTED_EDGE('',*,*,#17826,.F.);
#25859=ORIENTED_EDGE('',*,*,#17832,.T.);
#25860=ORIENTED_EDGE('',*,*,#17842,.T.);
#25861=ORIENTED_EDGE('',*,*,#17675,.T.);
#25862=ORIENTED_EDGE('',*,*,#17842,.F.);
#25863=ORIENTED_EDGE('',*,*,#17841,.T.);
#25864=ORIENTED_EDGE('',*,*,#17843,.T.);
#25865=ORIENTED_EDGE('',*,*,#17679,.T.);
#25866=ORIENTED_EDGE('',*,*,#17843,.F.);
#25867=ORIENTED_EDGE('',*,*,#17833,.T.);
#25868=ORIENTED_EDGE('',*,*,#17844,.T.);
#25869=ORIENTED_EDGE('',*,*,#17683,.T.);
#25870=ORIENTED_EDGE('',*,*,#17844,.F.);
#25871=ORIENTED_EDGE('',*,*,#17840,.T.);
#25872=ORIENTED_EDGE('',*,*,#17845,.T.);
#25873=ORIENTED_EDGE('',*,*,#17687,.T.);
#25874=ORIENTED_EDGE('',*,*,#17845,.F.);
#25875=ORIENTED_EDGE('',*,*,#17846,.T.);
#25876=ORIENTED_EDGE('',*,*,#17828,.T.);
#25877=ORIENTED_EDGE('',*,*,#17847,.T.);
#25878=ORIENTED_EDGE('',*,*,#17758,.T.);
#25879=ORIENTED_EDGE('',*,*,#17848,.T.);
#25880=ORIENTED_EDGE('',*,*,#17849,.T.);
#25881=ORIENTED_EDGE('',*,*,#17846,.F.);
#25882=ORIENTED_EDGE('',*,*,#17765,.T.);
#25883=ORIENTED_EDGE('',*,*,#17850,.T.);
#25884=ORIENTED_EDGE('',*,*,#17851,.T.);
#25885=ORIENTED_EDGE('',*,*,#17848,.F.);
#25886=ORIENTED_EDGE('',*,*,#17764,.T.);
#25887=ORIENTED_EDGE('',*,*,#17852,.T.);
#25888=ORIENTED_EDGE('',*,*,#17853,.T.);
#25889=ORIENTED_EDGE('',*,*,#17850,.F.);
#25890=ORIENTED_EDGE('',*,*,#17763,.T.);
#25891=ORIENTED_EDGE('',*,*,#17854,.T.);
#25892=ORIENTED_EDGE('',*,*,#17804,.T.);
#25893=ORIENTED_EDGE('',*,*,#17852,.F.);
#25894=ORIENTED_EDGE('',*,*,#17762,.T.);
#25895=ORIENTED_EDGE('',*,*,#17855,.T.);
#25896=ORIENTED_EDGE('',*,*,#17856,.T.);
#25897=ORIENTED_EDGE('',*,*,#17854,.F.);
#25898=ORIENTED_EDGE('',*,*,#17761,.T.);
#25899=ORIENTED_EDGE('',*,*,#17857,.T.);
#25900=ORIENTED_EDGE('',*,*,#17858,.T.);
#25901=ORIENTED_EDGE('',*,*,#17855,.F.);
#25902=ORIENTED_EDGE('',*,*,#17760,.T.);
#25903=ORIENTED_EDGE('',*,*,#17847,.F.);
#25904=ORIENTED_EDGE('',*,*,#17859,.T.);
#25905=ORIENTED_EDGE('',*,*,#17857,.F.);
#25906=ORIENTED_EDGE('',*,*,#17759,.T.);
#25907=ORIENTED_EDGE('',*,*,#17856,.F.);
#25908=ORIENTED_EDGE('',*,*,#17860,.T.);
#25909=ORIENTED_EDGE('',*,*,#17861,.F.);
#25910=ORIENTED_EDGE('',*,*,#17805,.T.);
#25911=ORIENTED_EDGE('',*,*,#17858,.F.);
#25912=ORIENTED_EDGE('',*,*,#17862,.F.);
#25913=ORIENTED_EDGE('',*,*,#17863,.F.);
#25914=ORIENTED_EDGE('',*,*,#17860,.F.);
#25915=ORIENTED_EDGE('',*,*,#17859,.F.);
#25916=ORIENTED_EDGE('',*,*,#17831,.T.);
#25917=ORIENTED_EDGE('',*,*,#17864,.F.);
#25918=ORIENTED_EDGE('',*,*,#17862,.T.);
#25919=ORIENTED_EDGE('',*,*,#17839,.T.);
#25920=ORIENTED_EDGE('',*,*,#17865,.T.);
#25921=ORIENTED_EDGE('',*,*,#17825,.T.);
#25922=ORIENTED_EDGE('',*,*,#17865,.F.);
#25923=ORIENTED_EDGE('',*,*,#17810,.T.);
#25924=ORIENTED_EDGE('',*,*,#17866,.T.);
#25925=ORIENTED_EDGE('',*,*,#17800,.T.);
#25926=ORIENTED_EDGE('',*,*,#17866,.F.);
#25927=ORIENTED_EDGE('',*,*,#17834,.T.);
#25928=ORIENTED_EDGE('',*,*,#17867,.T.);
#25929=ORIENTED_EDGE('',*,*,#17797,.T.);
#25930=ORIENTED_EDGE('',*,*,#17867,.F.);
#25931=ORIENTED_EDGE('',*,*,#17815,.T.);
#25932=ORIENTED_EDGE('',*,*,#17868,.T.);
#25933=ORIENTED_EDGE('',*,*,#17792,.T.);
#25934=ORIENTED_EDGE('',*,*,#17868,.F.);
#25935=ORIENTED_EDGE('',*,*,#17838,.T.);
#25936=ORIENTED_EDGE('',*,*,#17869,.T.);
#25937=ORIENTED_EDGE('',*,*,#17789,.T.);
#25938=ORIENTED_EDGE('',*,*,#17869,.F.);
#25939=ORIENTED_EDGE('',*,*,#17811,.T.);
#25940=ORIENTED_EDGE('',*,*,#17870,.T.);
#25941=ORIENTED_EDGE('',*,*,#17784,.T.);
#25942=ORIENTED_EDGE('',*,*,#17870,.F.);
#25943=ORIENTED_EDGE('',*,*,#17835,.T.);
#25944=ORIENTED_EDGE('',*,*,#17871,.T.);
#25945=ORIENTED_EDGE('',*,*,#17781,.T.);
#25946=ORIENTED_EDGE('',*,*,#17871,.F.);
#25947=ORIENTED_EDGE('',*,*,#17814,.T.);
#25948=ORIENTED_EDGE('',*,*,#17872,.T.);
#25949=ORIENTED_EDGE('',*,*,#17776,.T.);
#25950=ORIENTED_EDGE('',*,*,#17872,.F.);
#25951=ORIENTED_EDGE('',*,*,#17837,.T.);
#25952=ORIENTED_EDGE('',*,*,#17873,.T.);
#25953=ORIENTED_EDGE('',*,*,#17691,.T.);
#25954=ORIENTED_EDGE('',*,*,#17873,.F.);
#25955=ORIENTED_EDGE('',*,*,#17812,.T.);
#25956=ORIENTED_EDGE('',*,*,#17874,.T.);
#25957=ORIENTED_EDGE('',*,*,#17768,.T.);
#25958=ORIENTED_EDGE('',*,*,#17874,.F.);
#25959=ORIENTED_EDGE('',*,*,#17836,.T.);
#25960=ORIENTED_EDGE('',*,*,#17875,.T.);
#25961=ORIENTED_EDGE('',*,*,#17695,.T.);
#25962=ORIENTED_EDGE('',*,*,#17875,.F.);
#25963=ORIENTED_EDGE('',*,*,#17813,.T.);
#25964=ORIENTED_EDGE('',*,*,#17876,.T.);
#25965=ORIENTED_EDGE('',*,*,#17772,.T.);
#25966=ORIENTED_EDGE('',*,*,#17876,.F.);
#25967=ORIENTED_EDGE('',*,*,#17877,.T.);
#25968=ORIENTED_EDGE('',*,*,#17878,.T.);
#25969=ORIENTED_EDGE('',*,*,#17879,.T.);
#25970=ORIENTED_EDGE('',*,*,#17880,.T.);
#25971=ORIENTED_EDGE('',*,*,#17877,.F.);
#25972=ORIENTED_EDGE('',*,*,#17881,.T.);
#25973=ORIENTED_EDGE('',*,*,#17882,.T.);
#25974=ORIENTED_EDGE('',*,*,#17883,.T.);
#25975=ORIENTED_EDGE('',*,*,#17884,.T.);
#25976=ORIENTED_EDGE('',*,*,#17885,.T.);
#25977=ORIENTED_EDGE('',*,*,#17882,.F.);
#25978=ORIENTED_EDGE('',*,*,#17886,.T.);
#25979=ORIENTED_EDGE('',*,*,#17884,.F.);
#25980=ORIENTED_EDGE('',*,*,#17887,.T.);
#25981=ORIENTED_EDGE('',*,*,#17888,.T.);
#25982=ORIENTED_EDGE('',*,*,#17830,.T.);
#25983=ORIENTED_EDGE('',*,*,#17889,.T.);
#25984=ORIENTED_EDGE('',*,*,#17864,.T.);
#25985=ORIENTED_EDGE('',*,*,#17888,.F.);
#25986=ORIENTED_EDGE('',*,*,#17890,.T.);
#25987=ORIENTED_EDGE('',*,*,#17889,.F.);
#25988=ORIENTED_EDGE('',*,*,#17891,.T.);
#25989=ORIENTED_EDGE('',*,*,#17892,.T.);
#25990=ORIENTED_EDGE('',*,*,#17863,.T.);
#25991=ORIENTED_EDGE('',*,*,#17893,.T.);
#25992=ORIENTED_EDGE('',*,*,#17861,.T.);
#25993=ORIENTED_EDGE('',*,*,#17892,.F.);
#25994=ORIENTED_EDGE('',*,*,#17894,.T.);
#25995=ORIENTED_EDGE('',*,*,#17893,.F.);
#25996=ORIENTED_EDGE('',*,*,#17895,.T.);
#25997=ORIENTED_EDGE('',*,*,#17879,.F.);
#25998=ORIENTED_EDGE('',*,*,#17806,.T.);
#25999=ORIENTED_EDGE('',*,*,#17853,.F.);
#26000=ORIENTED_EDGE('',*,*,#17807,.T.);
#26001=ORIENTED_EDGE('',*,*,#17878,.F.);
#26002=ORIENTED_EDGE('',*,*,#17896,.T.);
#26003=ORIENTED_EDGE('',*,*,#17880,.F.);
#26004=ORIENTED_EDGE('',*,*,#17895,.F.);
#26005=ORIENTED_EDGE('',*,*,#17894,.F.);
#26006=ORIENTED_EDGE('',*,*,#17891,.F.);
#26007=ORIENTED_EDGE('',*,*,#17890,.F.);
#26008=ORIENTED_EDGE('',*,*,#17887,.F.);
#26009=ORIENTED_EDGE('',*,*,#17886,.F.);
#26010=ORIENTED_EDGE('',*,*,#17881,.F.);
#26011=ORIENTED_EDGE('',*,*,#17897,.F.);
#26012=ORIENTED_EDGE('',*,*,#17898,.F.);
#26013=ORIENTED_EDGE('',*,*,#17899,.F.);
#26014=ORIENTED_EDGE('',*,*,#17900,.F.);
#26015=ORIENTED_EDGE('',*,*,#17901,.F.);
#26016=ORIENTED_EDGE('',*,*,#17902,.F.);
#26017=ORIENTED_EDGE('',*,*,#17903,.F.);
#26018=ORIENTED_EDGE('',*,*,#17904,.F.);
#26019=ORIENTED_EDGE('',*,*,#17905,.T.);
#26020=ORIENTED_EDGE('',*,*,#17906,.T.);
#26021=ORIENTED_EDGE('',*,*,#17907,.T.);
#26022=ORIENTED_EDGE('',*,*,#17897,.T.);
#26023=ORIENTED_EDGE('',*,*,#17905,.F.);
#26024=ORIENTED_EDGE('',*,*,#17904,.T.);
#26025=ORIENTED_EDGE('',*,*,#17908,.T.);
#26026=ORIENTED_EDGE('',*,*,#17909,.T.);
#26027=ORIENTED_EDGE('',*,*,#17910,.T.);
#26028=ORIENTED_EDGE('',*,*,#17911,.T.);
#26029=ORIENTED_EDGE('',*,*,#17908,.F.);
#26030=ORIENTED_EDGE('',*,*,#17903,.T.);
#26031=ORIENTED_EDGE('',*,*,#17910,.F.);
#26032=ORIENTED_EDGE('',*,*,#17902,.T.);
#26033=ORIENTED_EDGE('',*,*,#17912,.T.);
#26034=ORIENTED_EDGE('',*,*,#17701,.T.);
#26035=ORIENTED_EDGE('',*,*,#17913,.T.);
#26036=ORIENTED_EDGE('',*,*,#17757,.T.);
#26037=ORIENTED_EDGE('',*,*,#17912,.F.);
#26038=ORIENTED_EDGE('',*,*,#17901,.T.);
#26039=ORIENTED_EDGE('',*,*,#17913,.F.);
#26040=ORIENTED_EDGE('',*,*,#17900,.T.);
#26041=ORIENTED_EDGE('',*,*,#17914,.T.);
#26042=ORIENTED_EDGE('',*,*,#17756,.T.);
#26043=ORIENTED_EDGE('',*,*,#17915,.T.);
#26044=ORIENTED_EDGE('',*,*,#17754,.T.);
#26045=ORIENTED_EDGE('',*,*,#17914,.F.);
#26046=ORIENTED_EDGE('',*,*,#17899,.T.);
#26047=ORIENTED_EDGE('',*,*,#17915,.F.);
#26048=ORIENTED_EDGE('',*,*,#17898,.T.);
#26049=ORIENTED_EDGE('',*,*,#17907,.F.);
#26050=ORIENTED_EDGE('',*,*,#17658,.T.);
#26051=ORIENTED_EDGE('',*,*,#17741,.F.);
#26052=ORIENTED_EDGE('',*,*,#17659,.T.);
#26053=ORIENTED_EDGE('',*,*,#17906,.F.);
#26054=ORIENTED_EDGE('',*,*,#17916,.T.);
#26055=ORIENTED_EDGE('',*,*,#17735,.F.);
#26056=ORIENTED_EDGE('',*,*,#17917,.T.);
#26057=ORIENTED_EDGE('',*,*,#17911,.F.);
#26058=ORIENTED_EDGE('',*,*,#17700,.T.);
#26059=ORIENTED_EDGE('',*,*,#17738,.F.);
#26060=ORIENTED_EDGE('',*,*,#17916,.F.);
#26061=ORIENTED_EDGE('',*,*,#17909,.F.);
#26062=ORIENTED_EDGE('',*,*,#17917,.F.);
#26063=ORIENTED_EDGE('',*,*,#17851,.F.);
#26064=ORIENTED_EDGE('',*,*,#17896,.F.);
#26065=ORIENTED_EDGE('',*,*,#17883,.F.);
#26066=ORIENTED_EDGE('',*,*,#17918,.F.);
#26067=ORIENTED_EDGE('',*,*,#17849,.F.);
#26068=ORIENTED_EDGE('',*,*,#17918,.T.);
#26069=ORIENTED_EDGE('',*,*,#17885,.F.);
#26070=ORIENTED_EDGE('',*,*,#17829,.T.);
#26853=PLANE('',#30557);
#26854=PLANE('',#30597);
#26855=PLANE('',#30626);
#26856=PLANE('',#30630);
#26857=PLANE('',#30634);
#26858=PLANE('',#30638);
#26859=PLANE('',#30644);
#26860=PLANE('',#30647);
#26861=PLANE('',#30690);
#26862=PLANE('',#30711);
#26863=PLANE('',#30726);
#26864=PLANE('',#30729);
#26865=PLANE('',#30732);
#26866=PLANE('',#30735);
#26867=PLANE('',#30740);
#26868=PLANE('',#30758);
#26869=PLANE('',#30762);
#26870=PLANE('',#30765);
#26871=PLANE('',#30768);
#26872=PLANE('',#30770);
#26873=PLANE('',#30777);
#26874=PLANE('',#30780);
#26875=PLANE('',#30782);
#26876=PLANE('',#30784);
#26877=PLANE('',#30787);
#26878=PLANE('',#30788);
#28343=ADVANCED_FACE('',(#4435),#2911,.F.);
#28344=ADVANCED_FACE('',(#4436,#1999,#2000,#2001,#2002,#2003,#2004,#2005,
#2006,#2007,#2008,#2009),#26853,.T.);
#28345=ADVANCED_FACE('',(#4437),#1844,.F.);
#28346=ADVANCED_FACE('',(#4438),#2912,.F.);
#28347=ADVANCED_FACE('',(#4439),#1845,.F.);
#28348=ADVANCED_FACE('',(#4440),#2913,.F.);
#28349=ADVANCED_FACE('',(#4441),#1846,.F.);
#28350=ADVANCED_FACE('',(#4442),#2914,.F.);
#28351=ADVANCED_FACE('',(#4443),#1847,.F.);
#28352=ADVANCED_FACE('',(#4444),#2915,.F.);
#28353=ADVANCED_FACE('',(#4445),#1848,.F.);
#28354=ADVANCED_FACE('',(#4446),#2916,.F.);
#28355=ADVANCED_FACE('',(#4447),#1849,.F.);
#28356=ADVANCED_FACE('',(#4448),#2917,.F.);
#28357=ADVANCED_FACE('',(#4449),#1850,.F.);
#28358=ADVANCED_FACE('',(#4450),#2918,.F.);
#28359=ADVANCED_FACE('',(#4451,#2010,#2011,#2012,#2013,#2014,#2015,#2016,
#2017,#2018,#2019,#2020),#26854,.T.);
#28360=ADVANCED_FACE('',(#4452),#1851,.F.);
#28361=ADVANCED_FACE('',(#4453),#2919,.F.);
#28362=ADVANCED_FACE('',(#4454),#1852,.F.);
#28363=ADVANCED_FACE('',(#4455),#2920,.F.);
#28364=ADVANCED_FACE('',(#4456),#1853,.F.);
#28365=ADVANCED_FACE('',(#4457),#2921,.F.);
#28366=ADVANCED_FACE('',(#4458),#1854,.F.);
#28367=ADVANCED_FACE('',(#4459),#2922,.F.);
#28368=ADVANCED_FACE('',(#4460),#1855,.F.);
#28369=ADVANCED_FACE('',(#4461),#26855,.T.);
#28370=ADVANCED_FACE('',(#4462),#2923,.F.);
#28371=ADVANCED_FACE('',(#4463),#26856,.T.);
#28372=ADVANCED_FACE('',(#4464),#2924,.F.);
#28373=ADVANCED_FACE('',(#4465),#26857,.T.);
#28374=ADVANCED_FACE('',(#4466),#2925,.F.);
#28375=ADVANCED_FACE('',(#4467),#26858,.T.);
#28376=ADVANCED_FACE('',(#4468),#2926,.F.);
#28377=ADVANCED_FACE('',(#4469),#1856,.F.);
#28378=ADVANCED_FACE('',(#4470),#26859,.T.);
#28379=ADVANCED_FACE('',(#4471),#1857,.F.);
#28380=ADVANCED_FACE('',(#4472,#2021),#26860,.F.);
#28381=ADVANCED_FACE('',(#4473),#2927,.F.);
#28382=ADVANCED_FACE('',(#4474),#1858,.F.);
#28383=ADVANCED_FACE('',(#4475),#2928,.F.);
#28384=ADVANCED_FACE('',(#4476),#1859,.F.);
#28385=ADVANCED_FACE('',(#4477),#2929,.F.);
#28386=ADVANCED_FACE('',(#4478),#1860,.F.);
#28387=ADVANCED_FACE('',(#4479),#2930,.F.);
#28388=ADVANCED_FACE('',(#4480),#1861,.F.);
#28389=ADVANCED_FACE('',(#4481),#2931,.F.);
#28390=ADVANCED_FACE('',(#4482),#1862,.F.);
#28391=ADVANCED_FACE('',(#4483),#2932,.F.);
#28392=ADVANCED_FACE('',(#4484),#1863,.F.);
#28393=ADVANCED_FACE('',(#4485),#2933,.F.);
#28394=ADVANCED_FACE('',(#4486),#1864,.F.);
#28395=ADVANCED_FACE('',(#4487),#2934,.F.);
#28396=ADVANCED_FACE('',(#4488),#1865,.F.);
#28397=ADVANCED_FACE('',(#4489),#2935,.F.);
#28398=ADVANCED_FACE('',(#4490),#1866,.F.);
#28399=ADVANCED_FACE('',(#4491),#2936,.F.);
#28400=ADVANCED_FACE('',(#4492,#2022,#2023,#2024,#2025,#2026,#2027,#2028,
#2029,#2030,#2031,#2032),#26861,.T.);
#28401=ADVANCED_FACE('',(#4493),#2937,.F.);
#28402=ADVANCED_FACE('',(#4494),#2938,.F.);
#28403=ADVANCED_FACE('',(#4495),#2939,.F.);
#28404=ADVANCED_FACE('',(#4496),#2940,.F.);
#28405=ADVANCED_FACE('',(#4497),#2941,.F.);
#28406=ADVANCED_FACE('',(#4498),#1867,.F.);
#28407=ADVANCED_FACE('',(#4499),#2942,.F.);
#28408=ADVANCED_FACE('',(#4500,#2033,#2034,#2035,#2036,#2037,#2038,#2039,
#2040,#2041,#2042,#2043),#26862,.T.);
#28409=ADVANCED_FACE('',(#4501),#2943,.F.);
#28410=ADVANCED_FACE('',(#4502),#2944,.F.);
#28411=ADVANCED_FACE('',(#4503),#2945,.F.);
#28412=ADVANCED_FACE('',(#4504),#2946,.F.);
#28413=ADVANCED_FACE('',(#4505),#26863,.T.);
#28414=ADVANCED_FACE('',(#4506),#2947,.T.);
#28415=ADVANCED_FACE('',(#4507),#26864,.T.);
#28416=ADVANCED_FACE('',(#4508),#2948,.T.);
#28417=ADVANCED_FACE('',(#4509),#26865,.T.);
#28418=ADVANCED_FACE('',(#4510),#2949,.T.);
#28419=ADVANCED_FACE('',(#4511),#26866,.T.);
#28420=ADVANCED_FACE('',(#4512),#2950,.T.);
#28421=ADVANCED_FACE('',(#4513),#1868,.T.);
#28422=ADVANCED_FACE('',(#4514),#26867,.T.);
#28423=ADVANCED_FACE('',(#4515),#1869,.T.);
#28424=ADVANCED_FACE('',(#4516),#2951,.F.);
#28425=ADVANCED_FACE('',(#4517),#2952,.F.);
#28426=ADVANCED_FACE('',(#4518),#2953,.F.);
#28427=ADVANCED_FACE('',(#4519),#2954,.F.);
#28428=ADVANCED_FACE('',(#4520),#2955,.F.);
#28429=ADVANCED_FACE('',(#4521),#2956,.F.);
#28430=ADVANCED_FACE('',(#4522),#2957,.F.);
#28431=ADVANCED_FACE('',(#4523),#2958,.F.);
#28432=ADVANCED_FACE('',(#4524),#2959,.F.);
#28433=ADVANCED_FACE('',(#4525),#2960,.F.);
#28434=ADVANCED_FACE('',(#4526),#2961,.F.);
#28435=ADVANCED_FACE('',(#4527),#2962,.F.);
#28436=ADVANCED_FACE('',(#4528),#2963,.T.);
#28437=ADVANCED_FACE('',(#4529),#26868,.T.);
#28438=ADVANCED_FACE('',(#4530),#2964,.T.);
#28439=ADVANCED_FACE('',(#4531),#26869,.T.);
#28440=ADVANCED_FACE('',(#4532),#2965,.T.);
#28441=ADVANCED_FACE('',(#4533),#26870,.T.);
#28442=ADVANCED_FACE('',(#4534),#2966,.T.);
#28443=ADVANCED_FACE('',(#4535),#26871,.T.);
#28444=ADVANCED_FACE('',(#4536),#1870,.T.);
#28445=ADVANCED_FACE('',(#4537,#2044),#26872,.T.);
#28446=ADVANCED_FACE('',(#4538),#2967,.F.);
#28447=ADVANCED_FACE('',(#4539),#26873,.T.);
#28448=ADVANCED_FACE('',(#4540),#2968,.F.);
#28449=ADVANCED_FACE('',(#4541),#26874,.T.);
#28450=ADVANCED_FACE('',(#4542),#2969,.F.);
#28451=ADVANCED_FACE('',(#4543),#26875,.T.);
#28452=ADVANCED_FACE('',(#4544),#2970,.F.);
#28453=ADVANCED_FACE('',(#4545),#26876,.T.);
#28454=ADVANCED_FACE('',(#4546),#1871,.F.);
#28455=ADVANCED_FACE('',(#4547),#1872,.F.);
#28456=ADVANCED_FACE('',(#4548),#26877,.T.);
#28457=ADVANCED_FACE('',(#4549),#26878,.T.);
#28458=ADVANCED_FACE('',(#4550),#1873,.T.);
#28477=CLOSED_SHELL('',(#28343,#28344,#28345,#28346,#28347,#28348,#28349,
#28350,#28351,#28352,#28353,#28354,#28355,#28356,#28357,#28358,#28359,#28360,
#28361,#28362,#28363,#28364,#28365,#28366,#28367,#28368,#28369,#28370,#28371,
#28372,#28373,#28374,#28375,#28376,#28377,#28378,#28379,#28380,#28381,#28382,
#28383,#28384,#28385,#28386,#28387,#28388,#28389,#28390,#28391,#28392,#28393,
#28394,#28395,#28396,#28397,#28398,#28399,#28400,#28401,#28402,#28403,#28404,
#28405,#28406,#28407,#28408,#28409,#28410,#28411,#28412,#28413,#28414,#28415,
#28416,#28417,#28418,#28419,#28420,#28421,#28422,#28423,#28424,#28425,#28426,
#28427,#28428,#28429,#28430,#28431,#28432,#28433,#28434,#28435,#28436,#28437,
#28438,#28439,#28440,#28441,#28442,#28443,#28444,#28445,#28446,#28447,#28448,
#28449,#28450,#28451,#28452,#28453,#28454,#28455,#28456,#28457,#28458));
#30553=AXIS2_PLACEMENT_3D('',#70851,#36927,#36928);
#30554=AXIS2_PLACEMENT_3D('',#70852,#36929,#36930);
#30555=AXIS2_PLACEMENT_3D('',#70854,#36931,#36932);
#30556=AXIS2_PLACEMENT_3D('',#70857,#36934,#36935);
#30557=AXIS2_PLACEMENT_3D('',#70858,#36936,#36937);
#30558=AXIS2_PLACEMENT_3D('',#70868,#36942,#36943);
#30559=AXIS2_PLACEMENT_3D('',#70870,#36944,#36945);
#30560=AXIS2_PLACEMENT_3D('',#70872,#36946,#36947);
#30561=AXIS2_PLACEMENT_3D('',#70874,#36948,#36949);
#30562=AXIS2_PLACEMENT_3D('',#70876,#36950,#36951);
#30563=AXIS2_PLACEMENT_3D('',#70878,#36952,#36953);
#30564=AXIS2_PLACEMENT_3D('',#70880,#36954,#36955);
#30565=AXIS2_PLACEMENT_3D('',#70882,#36956,#36957);
#30566=AXIS2_PLACEMENT_3D('',#70884,#36958,#36959);
#30567=AXIS2_PLACEMENT_3D('',#70886,#36960,#36961);
#30568=AXIS2_PLACEMENT_3D('',#70887,#36962,#36963);
#30569=AXIS2_PLACEMENT_3D('',#70890,#36965,#36966);
#30570=AXIS2_PLACEMENT_3D('',#70891,#36967,#36968);
#30571=AXIS2_PLACEMENT_3D('',#70894,#36970,#36971);
#30572=AXIS2_PLACEMENT_3D('',#70895,#36972,#36973);
#30573=AXIS2_PLACEMENT_3D('',#70898,#36975,#36976);
#30574=AXIS2_PLACEMENT_3D('',#70899,#36977,#36978);
#30575=AXIS2_PLACEMENT_3D('',#70902,#36980,#36981);
#30576=AXIS2_PLACEMENT_3D('',#70903,#36982,#36983);
#30577=AXIS2_PLACEMENT_3D('',#70906,#36985,#36986);
#30578=AXIS2_PLACEMENT_3D('',#70907,#36987,#36988);
#30579=AXIS2_PLACEMENT_3D('',#70910,#36990,#36991);
#30580=AXIS2_PLACEMENT_3D('',#70911,#36992,#36993);
#30581=AXIS2_PLACEMENT_3D('',#70914,#36995,#36996);
#30582=AXIS2_PLACEMENT_3D('',#70915,#36997,#36998);
#30583=AXIS2_PLACEMENT_3D('',#70918,#37000,#37001);
#30584=AXIS2_PLACEMENT_3D('',#70919,#37002,#37003);
#30585=AXIS2_PLACEMENT_3D('',#70922,#37005,#37006);
#30586=AXIS2_PLACEMENT_3D('',#70923,#37007,#37008);
#30587=AXIS2_PLACEMENT_3D('',#70926,#37010,#37011);
#30588=AXIS2_PLACEMENT_3D('',#70927,#37012,#37013);
#30589=AXIS2_PLACEMENT_3D('',#70930,#37015,#37016);
#30590=AXIS2_PLACEMENT_3D('',#70931,#37017,#37018);
#30591=AXIS2_PLACEMENT_3D('',#70934,#37020,#37021);
#30592=AXIS2_PLACEMENT_3D('',#70935,#37022,#37023);
#30593=AXIS2_PLACEMENT_3D('',#70938,#37025,#37026);
#30594=AXIS2_PLACEMENT_3D('',#70939,#37027,#37028);
#30595=AXIS2_PLACEMENT_3D('',#70941,#37029,#37030);
#30596=AXIS2_PLACEMENT_3D('',#70944,#37032,#37033);
#30597=AXIS2_PLACEMENT_3D('',#70945,#37034,#37035);
#30598=AXIS2_PLACEMENT_3D('',#70955,#37040,#37041);
#30599=AXIS2_PLACEMENT_3D('',#70957,#37042,#37043);
#30600=AXIS2_PLACEMENT_3D('',#70959,#37044,#37045);
#30601=AXIS2_PLACEMENT_3D('',#70961,#37046,#37047);
#30602=AXIS2_PLACEMENT_3D('',#70963,#37048,#37049);
#30603=AXIS2_PLACEMENT_3D('',#70965,#37050,#37051);
#30604=AXIS2_PLACEMENT_3D('',#70967,#37052,#37053);
#30605=AXIS2_PLACEMENT_3D('',#70969,#37054,#37055);
#30606=AXIS2_PLACEMENT_3D('',#70971,#37056,#37057);
#30607=AXIS2_PLACEMENT_3D('',#70973,#37058,#37059);
#30608=AXIS2_PLACEMENT_3D('',#70974,#37060,#37061);
#30609=AXIS2_PLACEMENT_3D('',#70976,#37062,#37063);
#30610=AXIS2_PLACEMENT_3D('',#70978,#37065,#37066);
#30611=AXIS2_PLACEMENT_3D('',#70981,#37068,#37069);
#30612=AXIS2_PLACEMENT_3D('',#70982,#37070,#37071);
#30613=AXIS2_PLACEMENT_3D('',#70984,#37072,#37073);
#30614=AXIS2_PLACEMENT_3D('',#70986,#37075,#37076);
#30615=AXIS2_PLACEMENT_3D('',#70989,#37078,#37079);
#30616=AXIS2_PLACEMENT_3D('',#70990,#37080,#37081);
#30617=AXIS2_PLACEMENT_3D('',#70992,#37082,#37083);
#30618=AXIS2_PLACEMENT_3D('',#70994,#37085,#37086);
#30619=AXIS2_PLACEMENT_3D('',#70997,#37088,#37089);
#30620=AXIS2_PLACEMENT_3D('',#70998,#37090,#37091);
#30621=AXIS2_PLACEMENT_3D('',#71000,#37092,#37093);
#30622=AXIS2_PLACEMENT_3D('',#71002,#37095,#37096);
#30623=AXIS2_PLACEMENT_3D('',#71005,#37098,#37099);
#30624=AXIS2_PLACEMENT_3D('',#71006,#37100,#37101);
#30625=AXIS2_PLACEMENT_3D('',#71008,#37102,#37103);
#30626=AXIS2_PLACEMENT_3D('',#71010,#37105,#37106);
#30627=AXIS2_PLACEMENT_3D('',#71016,#37110,#37111);
#30628=AXIS2_PLACEMENT_3D('',#71020,#37113,#37114);
#30629=AXIS2_PLACEMENT_3D('',#71021,#37115,#37116);
#30630=AXIS2_PLACEMENT_3D('',#71022,#37117,#37118);
#30631=AXIS2_PLACEMENT_3D('',#71028,#37122,#37123);
#30632=AXIS2_PLACEMENT_3D('',#71031,#37125,#37126);
#30633=AXIS2_PLACEMENT_3D('',#71032,#37127,#37128);
#30634=AXIS2_PLACEMENT_3D('',#71033,#37129,#37130);
#30635=AXIS2_PLACEMENT_3D('',#71037,#37133,#37134);
#30636=AXIS2_PLACEMENT_3D('',#71041,#37136,#37137);
#30637=AXIS2_PLACEMENT_3D('',#71042,#37138,#37139);
#30638=AXIS2_PLACEMENT_3D('',#71043,#37140,#37141);
#30639=AXIS2_PLACEMENT_3D('',#71049,#37145,#37146);
#30640=AXIS2_PLACEMENT_3D('',#71050,#37147,#37148);
#30641=AXIS2_PLACEMENT_3D('',#71051,#37149,#37150);
#30642=AXIS2_PLACEMENT_3D('',#71052,#37151,#37152);
#30643=AXIS2_PLACEMENT_3D('',#71055,#37154,#37155);
#30644=AXIS2_PLACEMENT_3D('',#71056,#37156,#37157);
#30645=AXIS2_PLACEMENT_3D('',#71060,#37160,#37161);
#30646=AXIS2_PLACEMENT_3D('',#71061,#37162,#37163);
#30647=AXIS2_PLACEMENT_3D('',#71062,#37164,#37165);
#30648=AXIS2_PLACEMENT_3D('',#71067,#37167,#37168);
#30649=AXIS2_PLACEMENT_3D('',#71071,#37170,#37171);
#30650=AXIS2_PLACEMENT_3D('',#71075,#37173,#37174);
#30651=AXIS2_PLACEMENT_3D('',#71078,#37176,#37177);
#30652=AXIS2_PLACEMENT_3D('',#71079,#37178,#37179);
#30653=AXIS2_PLACEMENT_3D('',#71082,#37181,#37182);
#30654=AXIS2_PLACEMENT_3D('',#71083,#37183,#37184);
#30655=AXIS2_PLACEMENT_3D('',#71085,#37185,#37186);
#30656=AXIS2_PLACEMENT_3D('',#71087,#37188,#37189);
#30657=AXIS2_PLACEMENT_3D('',#71090,#37191,#37192);
#30658=AXIS2_PLACEMENT_3D('',#71091,#37193,#37194);
#30659=AXIS2_PLACEMENT_3D('',#71093,#37195,#37196);
#30660=AXIS2_PLACEMENT_3D('',#71095,#37198,#37199);
#30661=AXIS2_PLACEMENT_3D('',#71098,#37201,#37202);
#30662=AXIS2_PLACEMENT_3D('',#71099,#37203,#37204);
#30663=AXIS2_PLACEMENT_3D('',#71101,#37205,#37206);
#30664=AXIS2_PLACEMENT_3D('',#71103,#37208,#37209);
#30665=AXIS2_PLACEMENT_3D('',#71106,#37211,#37212);
#30666=AXIS2_PLACEMENT_3D('',#71107,#37213,#37214);
#30667=AXIS2_PLACEMENT_3D('',#71110,#37216,#37217);
#30668=AXIS2_PLACEMENT_3D('',#71111,#37218,#37219);
#30669=AXIS2_PLACEMENT_3D('',#71114,#37221,#37222);
#30670=AXIS2_PLACEMENT_3D('',#71115,#37223,#37224);
#30671=AXIS2_PLACEMENT_3D('',#71117,#37225,#37226);
#30672=AXIS2_PLACEMENT_3D('',#71119,#37228,#37229);
#30673=AXIS2_PLACEMENT_3D('',#71122,#37231,#37232);
#30674=AXIS2_PLACEMENT_3D('',#71123,#37233,#37234);
#30675=AXIS2_PLACEMENT_3D('',#71126,#37236,#37237);
#30676=AXIS2_PLACEMENT_3D('',#71127,#37238,#37239);
#30677=AXIS2_PLACEMENT_3D('',#71130,#37241,#37242);
#30678=AXIS2_PLACEMENT_3D('',#71131,#37243,#37244);
#30679=AXIS2_PLACEMENT_3D('',#71133,#37245,#37246);
#30680=AXIS2_PLACEMENT_3D('',#71135,#37248,#37249);
#30681=AXIS2_PLACEMENT_3D('',#71138,#37251,#37252);
#30682=AXIS2_PLACEMENT_3D('',#71139,#37253,#37254);
#30683=AXIS2_PLACEMENT_3D('',#71142,#37256,#37257);
#30684=AXIS2_PLACEMENT_3D('',#71143,#37258,#37259);
#30685=AXIS2_PLACEMENT_3D('',#71146,#37261,#37262);
#30686=AXIS2_PLACEMENT_3D('',#71147,#37263,#37264);
#30687=AXIS2_PLACEMENT_3D('',#71149,#37265,#37266);
#30688=AXIS2_PLACEMENT_3D('',#71151,#37268,#37269);
#30689=AXIS2_PLACEMENT_3D('',#71153,#37270,#37271);
#30690=AXIS2_PLACEMENT_3D('',#71155,#37273,#37274);
#30691=AXIS2_PLACEMENT_3D('',#71165,#37279,#37280);
#30692=AXIS2_PLACEMENT_3D('',#71167,#37281,#37282);
#30693=AXIS2_PLACEMENT_3D('',#71169,#37283,#37284);
#30694=AXIS2_PLACEMENT_3D('',#71171,#37285,#37286);
#30695=AXIS2_PLACEMENT_3D('',#71173,#37287,#37288);
#30696=AXIS2_PLACEMENT_3D('',#71175,#37289,#37290);
#30697=AXIS2_PLACEMENT_3D('',#71177,#37291,#37292);
#30698=AXIS2_PLACEMENT_3D('',#71179,#37293,#37294);
#30699=AXIS2_PLACEMENT_3D('',#71181,#37295,#37296);
#30700=AXIS2_PLACEMENT_3D('',#71183,#37297,#37298);
#30701=AXIS2_PLACEMENT_3D('',#71184,#37299,#37300);
#30702=AXIS2_PLACEMENT_3D('',#71186,#37302,#37303);
#30703=AXIS2_PLACEMENT_3D('',#71188,#37305,#37306);
#30704=AXIS2_PLACEMENT_3D('',#71190,#37308,#37309);
#30705=AXIS2_PLACEMENT_3D('',#71192,#37311,#37312);
#30706=AXIS2_PLACEMENT_3D('',#71195,#37314,#37315);
#30707=AXIS2_PLACEMENT_3D('',#71196,#37316,#37317);
#30708=AXIS2_PLACEMENT_3D('',#71199,#37319,#37320);
#30709=AXIS2_PLACEMENT_3D('',#71200,#37321,#37322);
#30710=AXIS2_PLACEMENT_3D('',#71202,#37323,#37324);
#30711=AXIS2_PLACEMENT_3D('',#71204,#37326,#37327);
#30712=AXIS2_PLACEMENT_3D('',#71214,#37332,#37333);
#30713=AXIS2_PLACEMENT_3D('',#71216,#37334,#37335);
#30714=AXIS2_PLACEMENT_3D('',#71218,#37336,#37337);
#30715=AXIS2_PLACEMENT_3D('',#71220,#37338,#37339);
#30716=AXIS2_PLACEMENT_3D('',#71222,#37340,#37341);
#30717=AXIS2_PLACEMENT_3D('',#71224,#37342,#37343);
#30718=AXIS2_PLACEMENT_3D('',#71226,#37344,#37345);
#30719=AXIS2_PLACEMENT_3D('',#71228,#37346,#37347);
#30720=AXIS2_PLACEMENT_3D('',#71230,#37348,#37349);
#30721=AXIS2_PLACEMENT_3D('',#71232,#37350,#37351);
#30722=AXIS2_PLACEMENT_3D('',#71233,#37352,#37353);
#30723=AXIS2_PLACEMENT_3D('',#71235,#37355,#37356);
#30724=AXIS2_PLACEMENT_3D('',#71237,#37358,#37359);
#30725=AXIS2_PLACEMENT_3D('',#71239,#37361,#37362);
#30726=AXIS2_PLACEMENT_3D('',#71241,#37364,#37365);
#30727=AXIS2_PLACEMENT_3D('',#71244,#37368,#37369);
#30728=AXIS2_PLACEMENT_3D('',#71247,#37371,#37372);
#30729=AXIS2_PLACEMENT_3D('',#71248,#37373,#37374);
#30730=AXIS2_PLACEMENT_3D('',#71252,#37377,#37378);
#30731=AXIS2_PLACEMENT_3D('',#71254,#37380,#37381);
#30732=AXIS2_PLACEMENT_3D('',#71255,#37382,#37383);
#30733=AXIS2_PLACEMENT_3D('',#71257,#37385,#37386);
#30734=AXIS2_PLACEMENT_3D('',#71260,#37388,#37389);
#30735=AXIS2_PLACEMENT_3D('',#71261,#37390,#37391);
#30736=AXIS2_PLACEMENT_3D('',#71265,#37394,#37395);
#30737=AXIS2_PLACEMENT_3D('',#71266,#37396,#37397);
#30738=AXIS2_PLACEMENT_3D('',#71267,#37398,#37399);
#30739=AXIS2_PLACEMENT_3D('',#71270,#37401,#37402);
#30740=AXIS2_PLACEMENT_3D('',#71271,#37403,#37404);
#30741=AXIS2_PLACEMENT_3D('',#71275,#37407,#37408);
#30742=AXIS2_PLACEMENT_3D('',#71276,#37409,#37410);
#30743=AXIS2_PLACEMENT_3D('',#71277,#37411,#37412);
#30744=AXIS2_PLACEMENT_3D('',#71279,#37414,#37415);
#30745=AXIS2_PLACEMENT_3D('',#71281,#37417,#37418);
#30746=AXIS2_PLACEMENT_3D('',#71283,#37420,#37421);
#30747=AXIS2_PLACEMENT_3D('',#71285,#37423,#37424);
#30748=AXIS2_PLACEMENT_3D('',#71287,#37426,#37427);
#30749=AXIS2_PLACEMENT_3D('',#71289,#37429,#37430);
#30750=AXIS2_PLACEMENT_3D('',#71291,#37432,#37433);
#30751=AXIS2_PLACEMENT_3D('',#71293,#37435,#37436);
#30752=AXIS2_PLACEMENT_3D('',#71295,#37438,#37439);
#30753=AXIS2_PLACEMENT_3D('',#71297,#37441,#37442);
#30754=AXIS2_PLACEMENT_3D('',#71299,#37444,#37445);
#30755=AXIS2_PLACEMENT_3D('',#71301,#37447,#37448);
#30756=AXIS2_PLACEMENT_3D('',#71305,#37450,#37451);
#30757=AXIS2_PLACEMENT_3D('',#71308,#37453,#37454);
#30758=AXIS2_PLACEMENT_3D('',#71309,#37455,#37456);
#30759=AXIS2_PLACEMENT_3D('',#71315,#37460,#37461);
#30760=AXIS2_PLACEMENT_3D('',#71318,#37463,#37464);
#30761=AXIS2_PLACEMENT_3D('',#71319,#37465,#37466);
#30762=AXIS2_PLACEMENT_3D('',#71320,#37467,#37468);
#30763=AXIS2_PLACEMENT_3D('',#71324,#37471,#37472);
#30764=AXIS2_PLACEMENT_3D('',#71327,#37474,#37475);
#30765=AXIS2_PLACEMENT_3D('',#71328,#37476,#37477);
#30766=AXIS2_PLACEMENT_3D('',#71332,#37480,#37481);
#30767=AXIS2_PLACEMENT_3D('',#71335,#37483,#37484);
#30768=AXIS2_PLACEMENT_3D('',#71336,#37485,#37486);
#30769=AXIS2_PLACEMENT_3D('',#71338,#37488,#37489);
#30770=AXIS2_PLACEMENT_3D('',#71340,#37491,#37492);
#30771=AXIS2_PLACEMENT_3D('',#71343,#37493,#37494);
#30772=AXIS2_PLACEMENT_3D('',#71347,#37496,#37497);
#30773=AXIS2_PLACEMENT_3D('',#71351,#37499,#37500);
#30774=AXIS2_PLACEMENT_3D('',#71355,#37502,#37503);
#30775=AXIS2_PLACEMENT_3D('',#71357,#37505,#37506);
#30776=AXIS2_PLACEMENT_3D('',#71360,#37508,#37509);
#30777=AXIS2_PLACEMENT_3D('',#71362,#37511,#37512);
#30778=AXIS2_PLACEMENT_3D('',#71366,#37515,#37516);
#30779=AXIS2_PLACEMENT_3D('',#71368,#37518,#37519);
#30780=AXIS2_PLACEMENT_3D('',#71369,#37520,#37521);
#30781=AXIS2_PLACEMENT_3D('',#71371,#37523,#37524);
#30782=AXIS2_PLACEMENT_3D('',#71373,#37526,#37527);
#30783=AXIS2_PLACEMENT_3D('',#71375,#37529,#37530);
#30784=AXIS2_PLACEMENT_3D('',#71377,#37532,#37533);
#30785=AXIS2_PLACEMENT_3D('',#71378,#37534,#37535);
#30786=AXIS2_PLACEMENT_3D('',#71380,#37537,#37538);
#30787=AXIS2_PLACEMENT_3D('',#71382,#37540,#37541);
#30788=AXIS2_PLACEMENT_3D('',#71383,#37542,#37543);
#30789=AXIS2_PLACEMENT_3D('',#71385,#37545,#37546);
#36927=DIRECTION('axis',(0.,0.,1.));
#36928=DIRECTION('refdir',(1.,0.,0.));
#36929=DIRECTION('center_axis',(0.,-1.,0.));
#36930=DIRECTION('ref_axis',(1.,0.,0.));
#36931=DIRECTION('center_axis',(0.,-1.,0.));
#36932=DIRECTION('ref_axis',(1.,0.,0.));
#36933=DIRECTION('',(0.707106781186552,0.707106781186543,8.65956056235499E-17));
#36934=DIRECTION('center_axis',(0.,1.,0.));
#36935=DIRECTION('ref_axis',(1.,0.,0.));
#36936=DIRECTION('center_axis',(0.,-1.,0.));
#36937=DIRECTION('ref_axis',(1.,0.,0.));
#36938=DIRECTION('',(-1.,0.,0.));
#36939=DIRECTION('',(0.,0.,-1.));
#36940=DIRECTION('',(1.,0.,0.));
#36941=DIRECTION('',(0.,0.,1.));
#36942=DIRECTION('center_axis',(0.,-1.,0.));
#36943=DIRECTION('ref_axis',(1.,0.,0.));
#36944=DIRECTION('center_axis',(0.,-1.,0.));
#36945=DIRECTION('ref_axis',(1.,0.,0.));
#36946=DIRECTION('center_axis',(0.,-1.,0.));
#36947=DIRECTION('ref_axis',(1.,0.,0.));
#36948=DIRECTION('center_axis',(0.,-1.,0.));
#36949=DIRECTION('ref_axis',(1.,0.,0.));
#36950=DIRECTION('center_axis',(0.,-1.,0.));
#36951=DIRECTION('ref_axis',(1.,0.,0.));
#36952=DIRECTION('center_axis',(0.,-1.,0.));
#36953=DIRECTION('ref_axis',(1.,0.,0.));
#36954=DIRECTION('center_axis',(0.,-1.,0.));
#36955=DIRECTION('ref_axis',(1.,0.,0.));
#36956=DIRECTION('center_axis',(0.,-1.,0.));
#36957=DIRECTION('ref_axis',(1.,0.,0.));
#36958=DIRECTION('center_axis',(0.,-1.,0.));
#36959=DIRECTION('ref_axis',(1.,0.,0.));
#36960=DIRECTION('center_axis',(0.,-1.,0.));
#36961=DIRECTION('ref_axis',(1.,0.,0.));
#36962=DIRECTION('center_axis',(0.,1.,0.));
#36963=DIRECTION('ref_axis',(1.,0.,0.));
#36964=DIRECTION('',(0.,1.,0.));
#36965=DIRECTION('center_axis',(0.,-1.,0.));
#36966=DIRECTION('ref_axis',(1.,0.,0.));
#36967=DIRECTION('center_axis',(0.,-1.,0.));
#36968=DIRECTION('ref_axis',(1.,0.,0.));
#36969=DIRECTION('',(0.707106781186552,0.707106781186543,8.65956056235499E-17));
#36970=DIRECTION('center_axis',(0.,1.,0.));
#36971=DIRECTION('ref_axis',(1.,0.,0.));
#36972=DIRECTION('center_axis',(0.,1.,0.));
#36973=DIRECTION('ref_axis',(1.,0.,0.));
#36974=DIRECTION('',(0.,1.,0.));
#36975=DIRECTION('center_axis',(0.,-1.,0.));
#36976=DIRECTION('ref_axis',(1.,0.,0.));
#36977=DIRECTION('center_axis',(0.,-1.,0.));
#36978=DIRECTION('ref_axis',(1.,0.,0.));
#36979=DIRECTION('',(0.707106781186552,0.707106781186543,8.65956056235499E-17));
#36980=DIRECTION('center_axis',(0.,1.,0.));
#36981=DIRECTION('ref_axis',(1.,0.,0.));
#36982=DIRECTION('center_axis',(0.,1.,0.));
#36983=DIRECTION('ref_axis',(1.,0.,0.));
#36984=DIRECTION('',(0.,1.,0.));
#36985=DIRECTION('center_axis',(0.,-1.,0.));
#36986=DIRECTION('ref_axis',(1.,0.,0.));
#36987=DIRECTION('center_axis',(0.,-1.,0.));
#36988=DIRECTION('ref_axis',(1.,0.,0.));
#36989=DIRECTION('',(0.707106781186552,0.707106781186543,8.65956056235499E-17));
#36990=DIRECTION('center_axis',(0.,1.,0.));
#36991=DIRECTION('ref_axis',(1.,0.,0.));
#36992=DIRECTION('center_axis',(0.,1.,0.));
#36993=DIRECTION('ref_axis',(1.,0.,0.));
#36994=DIRECTION('',(0.,1.,0.));
#36995=DIRECTION('center_axis',(0.,-1.,0.));
#36996=DIRECTION('ref_axis',(1.,0.,0.));
#36997=DIRECTION('center_axis',(0.,-1.,0.));
#36998=DIRECTION('ref_axis',(1.,0.,0.));
#36999=DIRECTION('',(0.707106781186552,0.707106781186543,8.65956056235499E-17));
#37000=DIRECTION('center_axis',(0.,1.,0.));
#37001=DIRECTION('ref_axis',(1.,0.,0.));
#37002=DIRECTION('center_axis',(0.,1.,0.));
#37003=DIRECTION('ref_axis',(1.,0.,0.));
#37004=DIRECTION('',(0.,1.,0.));
#37005=DIRECTION('center_axis',(0.,-1.,0.));
#37006=DIRECTION('ref_axis',(1.,0.,0.));
#37007=DIRECTION('center_axis',(0.,-1.,0.));
#37008=DIRECTION('ref_axis',(1.,0.,0.));
#37009=DIRECTION('',(0.707106781186552,0.707106781186543,8.65956056235499E-17));
#37010=DIRECTION('center_axis',(0.,1.,0.));
#37011=DIRECTION('ref_axis',(1.,0.,0.));
#37012=DIRECTION('center_axis',(0.,1.,0.));
#37013=DIRECTION('ref_axis',(1.,0.,0.));
#37014=DIRECTION('',(0.,1.,0.));
#37015=DIRECTION('center_axis',(0.,-1.,0.));
#37016=DIRECTION('ref_axis',(1.,0.,0.));
#37017=DIRECTION('center_axis',(0.,-1.,0.));
#37018=DIRECTION('ref_axis',(1.,0.,0.));
#37019=DIRECTION('',(0.707106781186552,0.707106781186543,8.65956056235499E-17));
#37020=DIRECTION('center_axis',(0.,1.,0.));
#37021=DIRECTION('ref_axis',(1.,0.,0.));
#37022=DIRECTION('center_axis',(0.,1.,0.));
#37023=DIRECTION('ref_axis',(1.,0.,0.));
#37024=DIRECTION('',(0.,1.,0.));
#37025=DIRECTION('center_axis',(0.,-1.,0.));
#37026=DIRECTION('ref_axis',(1.,0.,0.));
#37027=DIRECTION('center_axis',(0.,1.,0.));
#37028=DIRECTION('ref_axis',(1.,0.,0.));
#37029=DIRECTION('center_axis',(0.,1.,0.));
#37030=DIRECTION('ref_axis',(1.,0.,0.));
#37031=DIRECTION('',(0.707106781186552,-0.707106781186543,-8.65956056235499E-17));
#37032=DIRECTION('center_axis',(0.,-1.,0.));
#37033=DIRECTION('ref_axis',(1.,0.,0.));
#37034=DIRECTION('center_axis',(0.,1.,0.));
#37035=DIRECTION('ref_axis',(-1.,0.,0.));
#37036=DIRECTION('',(1.,0.,0.));
#37037=DIRECTION('',(0.,0.,-1.));
#37038=DIRECTION('',(-1.,0.,0.));
#37039=DIRECTION('',(0.,0.,1.));
#37040=DIRECTION('center_axis',(0.,1.,0.));
#37041=DIRECTION('ref_axis',(1.,0.,0.));
#37042=DIRECTION('center_axis',(0.,1.,0.));
#37043=DIRECTION('ref_axis',(1.,0.,0.));
#37044=DIRECTION('center_axis',(0.,1.,0.));
#37045=DIRECTION('ref_axis',(1.,0.,0.));
#37046=DIRECTION('center_axis',(0.,1.,0.));
#37047=DIRECTION('ref_axis',(1.,0.,0.));
#37048=DIRECTION('center_axis',(0.,1.,0.));
#37049=DIRECTION('ref_axis',(1.,0.,0.));
#37050=DIRECTION('center_axis',(0.,1.,0.));
#37051=DIRECTION('ref_axis',(1.,0.,0.));
#37052=DIRECTION('center_axis',(0.,1.,0.));
#37053=DIRECTION('ref_axis',(1.,0.,0.));
#37054=DIRECTION('center_axis',(0.,1.,0.));
#37055=DIRECTION('ref_axis',(1.,0.,0.));
#37056=DIRECTION('center_axis',(0.,1.,0.));
#37057=DIRECTION('ref_axis',(1.,0.,0.));
#37058=DIRECTION('center_axis',(0.,1.,0.));
#37059=DIRECTION('ref_axis',(1.,0.,0.));
#37060=DIRECTION('center_axis',(0.,1.,0.));
#37061=DIRECTION('ref_axis',(1.,0.,0.));
#37062=DIRECTION('center_axis',(0.,1.,0.));
#37063=DIRECTION('ref_axis',(1.,0.,0.));
#37064=DIRECTION('',(0.,1.,0.));
#37065=DIRECTION('center_axis',(0.,1.,0.));
#37066=DIRECTION('ref_axis',(1.,0.,0.));
#37067=DIRECTION('',(0.707106781186552,-0.707106781186543,-8.65956056235499E-17));
#37068=DIRECTION('center_axis',(0.,-1.,0.));
#37069=DIRECTION('ref_axis',(1.,0.,0.));
#37070=DIRECTION('center_axis',(0.,1.,0.));
#37071=DIRECTION('ref_axis',(1.,0.,0.));
#37072=DIRECTION('center_axis',(0.,1.,0.));
#37073=DIRECTION('ref_axis',(1.,0.,0.));
#37074=DIRECTION('',(0.,1.,0.));
#37075=DIRECTION('center_axis',(0.,1.,0.));
#37076=DIRECTION('ref_axis',(1.,0.,0.));
#37077=DIRECTION('',(0.707106781186552,-0.707106781186543,-8.65956056235499E-17));
#37078=DIRECTION('center_axis',(0.,-1.,0.));
#37079=DIRECTION('ref_axis',(1.,0.,0.));
#37080=DIRECTION('center_axis',(0.,1.,0.));
#37081=DIRECTION('ref_axis',(1.,0.,0.));
#37082=DIRECTION('center_axis',(0.,1.,0.));
#37083=DIRECTION('ref_axis',(1.,0.,0.));
#37084=DIRECTION('',(0.,1.,0.));
#37085=DIRECTION('center_axis',(0.,1.,0.));
#37086=DIRECTION('ref_axis',(1.,0.,0.));
#37087=DIRECTION('',(0.707106781186552,-0.707106781186543,-8.65956056235499E-17));
#37088=DIRECTION('center_axis',(0.,-1.,0.));
#37089=DIRECTION('ref_axis',(1.,0.,0.));
#37090=DIRECTION('center_axis',(0.,1.,0.));
#37091=DIRECTION('ref_axis',(1.,0.,0.));
#37092=DIRECTION('center_axis',(0.,1.,0.));
#37093=DIRECTION('ref_axis',(1.,0.,0.));
#37094=DIRECTION('',(0.,1.,0.));
#37095=DIRECTION('center_axis',(0.,1.,0.));
#37096=DIRECTION('ref_axis',(1.,0.,0.));
#37097=DIRECTION('',(0.707106781186552,-0.707106781186543,-8.65956056235499E-17));
#37098=DIRECTION('center_axis',(0.,-1.,0.));
#37099=DIRECTION('ref_axis',(1.,0.,0.));
#37100=DIRECTION('center_axis',(0.,1.,0.));
#37101=DIRECTION('ref_axis',(1.,0.,0.));
#37102=DIRECTION('center_axis',(0.,1.,0.));
#37103=DIRECTION('ref_axis',(1.,0.,0.));
#37104=DIRECTION('',(0.,1.,0.));
#37105=DIRECTION('center_axis',(0.,0.707106781186548,-0.707106781186548));
#37106=DIRECTION('ref_axis',(-1.,0.,0.));
#37107=DIRECTION('',(0.,0.707106781186548,0.707106781186548));
#37108=DIRECTION('',(0.,-0.707106781186548,-0.707106781186548));
#37109=DIRECTION('',(-1.,0.,0.));
#37110=DIRECTION('center_axis',(0.,0.,-1.));
#37111=DIRECTION('ref_axis',(-0.707106781186553,-0.707106781186542,0.));
#37112=DIRECTION('',(0.707106781186565,0.,0.70710678118653));
#37113=DIRECTION('center_axis',(0.,0.,1.));
#37114=DIRECTION('ref_axis',(-0.707106781186553,-0.707106781186542,0.));
#37115=DIRECTION('center_axis',(0.,0.,-1.));
#37116=DIRECTION('ref_axis',(-0.707106781186553,-0.707106781186542,0.));
#37117=DIRECTION('center_axis',(0.707106781186543,0.,-0.707106781186552));
#37118=DIRECTION('ref_axis',(-0.707106781186552,0.,-0.707106781186543));
#37119=DIRECTION('',(0.707106781186552,0.,0.707106781186543));
#37120=DIRECTION('',(0.,-1.,0.));
#37121=DIRECTION('',(0.,1.,0.));
#37122=DIRECTION('center_axis',(0.,0.,-1.));
#37123=DIRECTION('ref_axis',(-0.707106781186544,0.707106781186551,0.));
#37124=DIRECTION('',(0.,-0.707106781186546,0.707106781186549));
#37125=DIRECTION('center_axis',(0.,0.,1.));
#37126=DIRECTION('ref_axis',(-0.707106781186544,0.707106781186551,0.));
#37127=DIRECTION('center_axis',(0.,0.,-1.));
#37128=DIRECTION('ref_axis',(-0.707106781186544,0.707106781186551,0.));
#37129=DIRECTION('center_axis',(0.,-0.707106781186548,-0.707106781186548));
#37130=DIRECTION('ref_axis',(-1.,0.,0.));
#37131=DIRECTION('',(0.,-0.707106781186548,0.707106781186548));
#37132=DIRECTION('',(1.,0.,0.));
#37133=DIRECTION('center_axis',(0.,0.,-1.));
#37134=DIRECTION('ref_axis',(0.707106781186544,0.707106781186551,0.));
#37135=DIRECTION('',(-0.707106781186577,0.,0.707106781186518));
#37136=DIRECTION('center_axis',(0.,0.,1.));
#37137=DIRECTION('ref_axis',(0.707106781186544,0.707106781186551,0.));
#37138=DIRECTION('center_axis',(0.,0.,-1.));
#37139=DIRECTION('ref_axis',(0.707106781186544,0.707106781186551,0.));
#37140=DIRECTION('center_axis',(-0.707106781186543,0.,-0.707106781186552));
#37141=DIRECTION('ref_axis',(-0.707106781186552,0.,0.707106781186543));
#37142=DIRECTION('',(-0.707106781186552,0.,0.707106781186543));
#37143=DIRECTION('',(0.,1.,0.));
#37144=DIRECTION('',(0.,-1.,0.));
#37145=DIRECTION('center_axis',(0.,0.,-1.));
#37146=DIRECTION('ref_axis',(0.707106781186544,-0.707106781186551,0.));
#37147=DIRECTION('center_axis',(0.,0.,1.));
#37148=DIRECTION('ref_axis',(0.707106781186544,-0.707106781186551,0.));
#37149=DIRECTION('center_axis',(0.,0.,-1.));
#37150=DIRECTION('ref_axis',(0.707106781186544,-0.707106781186551,0.));
#37151=DIRECTION('center_axis',(0.,0.,1.));
#37152=DIRECTION('ref_axis',(0.707106781186544,0.707106781186551,0.));
#37153=DIRECTION('',(0.,0.,1.));
#37154=DIRECTION('center_axis',(0.,0.,-1.));
#37155=DIRECTION('ref_axis',(0.707106781186544,0.707106781186551,0.));
#37156=DIRECTION('center_axis',(-1.,0.,0.));
#37157=DIRECTION('ref_axis',(0.,-1.,0.));
#37158=DIRECTION('',(0.,0.,-1.));
#37159=DIRECTION('',(0.,-1.,0.));
#37160=DIRECTION('center_axis',(0.,0.,1.));
#37161=DIRECTION('ref_axis',(0.707106781186544,-0.707106781186551,0.));
#37162=DIRECTION('center_axis',(0.,0.,-1.));
#37163=DIRECTION('ref_axis',(0.707106781186544,-0.707106781186551,0.));
#37164=DIRECTION('center_axis',(0.,0.,1.));
#37165=DIRECTION('ref_axis',(1.,0.,0.));
#37166=DIRECTION('',(-1.,0.,0.));
#37167=DIRECTION('center_axis',(0.,0.,1.));
#37168=DIRECTION('ref_axis',(0.707106781186546,0.707106781186549,0.));
#37169=DIRECTION('',(0.,1.,0.));
#37170=DIRECTION('center_axis',(0.,0.,1.));
#37171=DIRECTION('ref_axis',(0.707106781186546,-0.707106781186549,0.));
#37172=DIRECTION('',(1.,0.,0.));
#37173=DIRECTION('center_axis',(0.,0.,1.));
#37174=DIRECTION('ref_axis',(-0.707106781186546,-0.707106781186549,0.));
#37175=DIRECTION('',(0.,-1.,0.));
#37176=DIRECTION('center_axis',(0.,0.,1.));
#37177=DIRECTION('ref_axis',(-0.707106781186549,0.707106781186546,0.));
#37178=DIRECTION('center_axis',(0.,1.,0.));
#37179=DIRECTION('ref_axis',(1.,0.,0.));
#37180=DIRECTION('',(0.707106781186552,-0.707106781186543,-8.65956056235499E-17));
#37181=DIRECTION('center_axis',(0.,-1.,0.));
#37182=DIRECTION('ref_axis',(1.,0.,0.));
#37183=DIRECTION('center_axis',(0.,1.,0.));
#37184=DIRECTION('ref_axis',(1.,0.,0.));
#37185=DIRECTION('center_axis',(0.,1.,0.));
#37186=DIRECTION('ref_axis',(1.,0.,0.));
#37187=DIRECTION('',(0.,1.,0.));
#37188=DIRECTION('center_axis',(0.,1.,0.));
#37189=DIRECTION('ref_axis',(1.,0.,0.));
#37190=DIRECTION('',(0.707106781186552,-0.707106781186543,-8.65956056235499E-17));
#37191=DIRECTION('center_axis',(0.,-1.,0.));
#37192=DIRECTION('ref_axis',(1.,0.,0.));
#37193=DIRECTION('center_axis',(0.,1.,0.));
#37194=DIRECTION('ref_axis',(1.,0.,0.));
#37195=DIRECTION('center_axis',(0.,1.,0.));
#37196=DIRECTION('ref_axis',(1.,0.,0.));
#37197=DIRECTION('',(0.,1.,0.));
#37198=DIRECTION('center_axis',(0.,1.,0.));
#37199=DIRECTION('ref_axis',(1.,0.,0.));
#37200=DIRECTION('',(0.707106781186552,-0.707106781186543,-8.65956056235499E-17));
#37201=DIRECTION('center_axis',(0.,-1.,0.));
#37202=DIRECTION('ref_axis',(1.,0.,0.));
#37203=DIRECTION('center_axis',(0.,1.,0.));
#37204=DIRECTION('ref_axis',(1.,0.,0.));
#37205=DIRECTION('center_axis',(0.,1.,0.));
#37206=DIRECTION('ref_axis',(1.,0.,0.));
#37207=DIRECTION('',(0.,1.,0.));
#37208=DIRECTION('center_axis',(0.,-1.,0.));
#37209=DIRECTION('ref_axis',(1.,0.,0.));
#37210=DIRECTION('',(0.707106781186552,0.707106781186543,8.65956056235499E-17));
#37211=DIRECTION('center_axis',(0.,1.,0.));
#37212=DIRECTION('ref_axis',(1.,0.,0.));
#37213=DIRECTION('center_axis',(0.,1.,0.));
#37214=DIRECTION('ref_axis',(1.,0.,0.));
#37215=DIRECTION('',(0.,1.,0.));
#37216=DIRECTION('center_axis',(0.,-1.,0.));
#37217=DIRECTION('ref_axis',(1.,0.,0.));
#37218=DIRECTION('center_axis',(0.,1.,0.));
#37219=DIRECTION('ref_axis',(1.,0.,0.));
#37220=DIRECTION('',(0.707106781186552,-0.707106781186543,-8.65956056235499E-17));
#37221=DIRECTION('center_axis',(0.,-1.,0.));
#37222=DIRECTION('ref_axis',(1.,0.,0.));
#37223=DIRECTION('center_axis',(0.,1.,0.));
#37224=DIRECTION('ref_axis',(1.,0.,0.));
#37225=DIRECTION('center_axis',(0.,1.,0.));
#37226=DIRECTION('ref_axis',(1.,0.,0.));
#37227=DIRECTION('',(0.,1.,0.));
#37228=DIRECTION('center_axis',(0.,-1.,0.));
#37229=DIRECTION('ref_axis',(1.,0.,0.));
#37230=DIRECTION('',(0.707106781186552,0.707106781186543,8.65956056235499E-17));
#37231=DIRECTION('center_axis',(0.,1.,0.));
#37232=DIRECTION('ref_axis',(1.,0.,0.));
#37233=DIRECTION('center_axis',(0.,1.,0.));
#37234=DIRECTION('ref_axis',(1.,0.,0.));
#37235=DIRECTION('',(0.,1.,0.));
#37236=DIRECTION('center_axis',(0.,-1.,0.));
#37237=DIRECTION('ref_axis',(1.,0.,0.));
#37238=DIRECTION('center_axis',(0.,1.,0.));
#37239=DIRECTION('ref_axis',(1.,0.,0.));
#37240=DIRECTION('',(0.707106781186552,-0.707106781186543,-8.65956056235499E-17));
#37241=DIRECTION('center_axis',(0.,-1.,0.));
#37242=DIRECTION('ref_axis',(1.,0.,0.));
#37243=DIRECTION('center_axis',(0.,1.,0.));
#37244=DIRECTION('ref_axis',(1.,0.,0.));
#37245=DIRECTION('center_axis',(0.,1.,0.));
#37246=DIRECTION('ref_axis',(1.,0.,0.));
#37247=DIRECTION('',(0.,1.,0.));
#37248=DIRECTION('center_axis',(0.,-1.,0.));
#37249=DIRECTION('ref_axis',(1.,0.,0.));
#37250=DIRECTION('',(0.707106781186552,0.707106781186543,8.65956056235499E-17));
#37251=DIRECTION('center_axis',(0.,1.,0.));
#37252=DIRECTION('ref_axis',(1.,0.,0.));
#37253=DIRECTION('center_axis',(0.,1.,0.));
#37254=DIRECTION('ref_axis',(1.,0.,0.));
#37255=DIRECTION('',(0.,1.,0.));
#37256=DIRECTION('center_axis',(0.,-1.,0.));
#37257=DIRECTION('ref_axis',(1.,0.,0.));
#37258=DIRECTION('center_axis',(0.,1.,0.));
#37259=DIRECTION('ref_axis',(1.,0.,0.));
#37260=DIRECTION('',(0.707106781186552,-0.707106781186543,-8.65956056235499E-17));
#37261=DIRECTION('center_axis',(0.,-1.,0.));
#37262=DIRECTION('ref_axis',(1.,0.,0.));
#37263=DIRECTION('center_axis',(0.,1.,0.));
#37264=DIRECTION('ref_axis',(1.,0.,0.));
#37265=DIRECTION('center_axis',(0.,1.,0.));
#37266=DIRECTION('ref_axis',(1.,0.,0.));
#37267=DIRECTION('',(0.,1.,0.));
#37268=DIRECTION('center_axis',(0.,-1.,0.));
#37269=DIRECTION('ref_axis',(1.,0.,0.));
#37270=DIRECTION('center_axis',(0.,-1.,0.));
#37271=DIRECTION('ref_axis',(1.,0.,0.));
#37272=DIRECTION('',(0.707106781186552,0.707106781186543,8.65956056235499E-17));
#37273=DIRECTION('center_axis',(0.,-1.,0.));
#37274=DIRECTION('ref_axis',(1.,0.,0.));
#37275=DIRECTION('',(-1.,0.,0.));
#37276=DIRECTION('',(0.,0.,-1.));
#37277=DIRECTION('',(1.,0.,0.));
#37278=DIRECTION('',(0.,0.,1.));
#37279=DIRECTION('center_axis',(0.,-1.,0.));
#37280=DIRECTION('ref_axis',(1.,0.,0.));
#37281=DIRECTION('center_axis',(0.,-1.,0.));
#37282=DIRECTION('ref_axis',(1.,0.,0.));
#37283=DIRECTION('center_axis',(0.,-1.,0.));
#37284=DIRECTION('ref_axis',(1.,0.,0.));
#37285=DIRECTION('center_axis',(0.,-1.,0.));
#37286=DIRECTION('ref_axis',(1.,0.,0.));
#37287=DIRECTION('center_axis',(0.,-1.,0.));
#37288=DIRECTION('ref_axis',(1.,0.,0.));
#37289=DIRECTION('center_axis',(0.,-1.,0.));
#37290=DIRECTION('ref_axis',(1.,0.,0.));
#37291=DIRECTION('center_axis',(0.,-1.,0.));
#37292=DIRECTION('ref_axis',(1.,0.,0.));
#37293=DIRECTION('center_axis',(0.,-1.,0.));
#37294=DIRECTION('ref_axis',(1.,0.,0.));
#37295=DIRECTION('center_axis',(0.,-1.,0.));
#37296=DIRECTION('ref_axis',(1.,0.,0.));
#37297=DIRECTION('center_axis',(0.,-1.,0.));
#37298=DIRECTION('ref_axis',(1.,0.,0.));
#37299=DIRECTION('center_axis',(0.,-1.,0.));
#37300=DIRECTION('ref_axis',(1.,0.,0.));
#37301=DIRECTION('',(0.707106781186552,0.707106781186543,8.65956056235499E-17));
#37302=DIRECTION('center_axis',(0.,-1.,0.));
#37303=DIRECTION('ref_axis',(1.,0.,0.));
#37304=DIRECTION('',(0.707106781186552,0.707106781186543,8.65956056235499E-17));
#37305=DIRECTION('center_axis',(0.,-1.,0.));
#37306=DIRECTION('ref_axis',(1.,0.,0.));
#37307=DIRECTION('',(0.707106781186552,0.707106781186543,8.65956056235499E-17));
#37308=DIRECTION('center_axis',(0.,-1.,0.));
#37309=DIRECTION('ref_axis',(1.,0.,0.));
#37310=DIRECTION('',(0.707106781186552,0.707106781186543,8.65956056235499E-17));
#37311=DIRECTION('center_axis',(0.,-1.,0.));
#37312=DIRECTION('ref_axis',(1.,0.,0.));
#37313=DIRECTION('',(0.707106781186552,0.707106781186543,8.65956056235499E-17));
#37314=DIRECTION('center_axis',(0.,1.,0.));
#37315=DIRECTION('ref_axis',(1.,0.,0.));
#37316=DIRECTION('center_axis',(0.,1.,0.));
#37317=DIRECTION('ref_axis',(1.,0.,0.));
#37318=DIRECTION('',(0.,1.,0.));
#37319=DIRECTION('center_axis',(0.,-1.,0.));
#37320=DIRECTION('ref_axis',(1.,0.,0.));
#37321=DIRECTION('center_axis',(0.,1.,0.));
#37322=DIRECTION('ref_axis',(1.,0.,0.));
#37323=DIRECTION('center_axis',(0.,1.,0.));
#37324=DIRECTION('ref_axis',(1.,0.,0.));
#37325=DIRECTION('',(0.707106781186552,-0.707106781186543,-8.65956056235499E-17));
#37326=DIRECTION('center_axis',(0.,1.,0.));
#37327=DIRECTION('ref_axis',(-1.,0.,0.));
#37328=DIRECTION('',(1.,0.,0.));
#37329=DIRECTION('',(0.,0.,-1.));
#37330=DIRECTION('',(-1.,0.,0.));
#37331=DIRECTION('',(0.,0.,1.));
#37332=DIRECTION('center_axis',(0.,1.,0.));
#37333=DIRECTION('ref_axis',(1.,0.,0.));
#37334=DIRECTION('center_axis',(0.,1.,0.));
#37335=DIRECTION('ref_axis',(1.,0.,0.));
#37336=DIRECTION('center_axis',(0.,1.,0.));
#37337=DIRECTION('ref_axis',(1.,0.,0.));
#37338=DIRECTION('center_axis',(0.,1.,0.));
#37339=DIRECTION('ref_axis',(1.,0.,0.));
#37340=DIRECTION('center_axis',(0.,1.,0.));
#37341=DIRECTION('ref_axis',(1.,0.,0.));
#37342=DIRECTION('center_axis',(0.,1.,0.));
#37343=DIRECTION('ref_axis',(1.,0.,0.));
#37344=DIRECTION('center_axis',(0.,1.,0.));
#37345=DIRECTION('ref_axis',(1.,0.,0.));
#37346=DIRECTION('center_axis',(0.,1.,0.));
#37347=DIRECTION('ref_axis',(1.,0.,0.));
#37348=DIRECTION('center_axis',(0.,1.,0.));
#37349=DIRECTION('ref_axis',(1.,0.,0.));
#37350=DIRECTION('center_axis',(0.,1.,0.));
#37351=DIRECTION('ref_axis',(1.,0.,0.));
#37352=DIRECTION('center_axis',(0.,1.,0.));
#37353=DIRECTION('ref_axis',(1.,0.,0.));
#37354=DIRECTION('',(0.707106781186552,-0.707106781186543,-8.65956056235499E-17));
#37355=DIRECTION('center_axis',(0.,1.,0.));
#37356=DIRECTION('ref_axis',(1.,0.,0.));
#37357=DIRECTION('',(0.707106781186552,-0.707106781186543,-8.65956056235499E-17));
#37358=DIRECTION('center_axis',(0.,1.,0.));
#37359=DIRECTION('ref_axis',(1.,0.,0.));
#37360=DIRECTION('',(0.707106781186552,-0.707106781186543,-8.65956056235499E-17));
#37361=DIRECTION('center_axis',(0.,1.,0.));
#37362=DIRECTION('ref_axis',(1.,0.,0.));
#37363=DIRECTION('',(0.707106781186552,-0.707106781186543,-8.65956056235499E-17));
#37364=DIRECTION('center_axis',(0.,0.707106781186548,-0.707106781186548));
#37365=DIRECTION('ref_axis',(-1.,0.,0.));
#37366=DIRECTION('',(0.,0.707106781186548,0.707106781186548));
#37367=DIRECTION('',(0.,-0.707106781186548,-0.707106781186548));
#37368=DIRECTION('center_axis',(0.,0.,1.));
#37369=DIRECTION('ref_axis',(-0.707106781186549,0.707106781186546,0.));
#37370=DIRECTION('',(-0.707106781186552,0.,0.707106781186543));
#37371=DIRECTION('center_axis',(0.,0.,-1.));
#37372=DIRECTION('ref_axis',(-0.70710678118655,0.707106781186546,0.));
#37373=DIRECTION('center_axis',(-0.707106781186543,0.,-0.707106781186552));
#37374=DIRECTION('ref_axis',(-0.707106781186552,0.,0.707106781186543));
#37375=DIRECTION('',(-0.707106781186552,0.,0.707106781186543));
#37376=DIRECTION('',(0.,1.,0.));
#37377=DIRECTION('center_axis',(0.,0.,1.));
#37378=DIRECTION('ref_axis',(-0.707106781186546,-0.707106781186549,0.));
#37379=DIRECTION('',(0.,-0.707106781186544,0.707106781186551));
#37380=DIRECTION('center_axis',(0.,0.,-1.));
#37381=DIRECTION('ref_axis',(-0.707106781186546,-0.707106781186549,0.));
#37382=DIRECTION('center_axis',(0.,-0.707106781186548,-0.707106781186548));
#37383=DIRECTION('ref_axis',(-1.,0.,0.));
#37384=DIRECTION('',(0.,-0.707106781186548,0.707106781186548));
#37385=DIRECTION('center_axis',(0.,0.,1.));
#37386=DIRECTION('ref_axis',(0.707106781186546,-0.707106781186549,0.));
#37387=DIRECTION('',(0.707106781186552,0.,0.707106781186543));
#37388=DIRECTION('center_axis',(0.,0.,-1.));
#37389=DIRECTION('ref_axis',(0.707106781186546,-0.707106781186549,0.));
#37390=DIRECTION('center_axis',(0.707106781186543,0.,-0.707106781186552));
#37391=DIRECTION('ref_axis',(-0.707106781186552,0.,-0.707106781186543));
#37392=DIRECTION('',(0.707106781186552,0.,0.707106781186543));
#37393=DIRECTION('',(0.,-1.,0.));
#37394=DIRECTION('center_axis',(0.,0.,1.));
#37395=DIRECTION('ref_axis',(0.707106781186546,0.707106781186549,0.));
#37396=DIRECTION('center_axis',(0.,0.,-1.));
#37397=DIRECTION('ref_axis',(0.707106781186546,0.707106781186549,0.));
#37398=DIRECTION('center_axis',(0.,0.,1.));
#37399=DIRECTION('ref_axis',(0.707106781186546,-0.707106781186549,0.));
#37400=DIRECTION('',(0.,0.,1.));
#37401=DIRECTION('center_axis',(0.,0.,1.));
#37402=DIRECTION('ref_axis',(0.707106781186546,-0.707106781186549,0.));
#37403=DIRECTION('center_axis',(1.,0.,0.));
#37404=DIRECTION('ref_axis',(0.,1.,0.));
#37405=DIRECTION('',(0.,0.,-1.));
#37406=DIRECTION('',(0.,1.,0.));
#37407=DIRECTION('center_axis',(0.,0.,1.));
#37408=DIRECTION('ref_axis',(0.707106781186546,0.707106781186549,0.));
#37409=DIRECTION('center_axis',(0.,0.,1.));
#37410=DIRECTION('ref_axis',(0.707106781186546,0.707106781186549,0.));
#37411=DIRECTION('center_axis',(0.,1.,0.));
#37412=DIRECTION('ref_axis',(1.,0.,0.));
#37413=DIRECTION('',(0.707106781186552,-0.707106781186543,-8.65956056235499E-17));
#37414=DIRECTION('center_axis',(0.,-1.,0.));
#37415=DIRECTION('ref_axis',(1.,0.,0.));
#37416=DIRECTION('',(0.707106781186552,0.707106781186543,8.65956056235499E-17));
#37417=DIRECTION('center_axis',(0.,1.,0.));
#37418=DIRECTION('ref_axis',(1.,0.,0.));
#37419=DIRECTION('',(0.707106781186552,-0.707106781186543,-8.65956056235499E-17));
#37420=DIRECTION('center_axis',(0.,-1.,0.));
#37421=DIRECTION('ref_axis',(1.,0.,0.));
#37422=DIRECTION('',(0.707106781186552,0.707106781186543,8.65956056235499E-17));
#37423=DIRECTION('center_axis',(0.,1.,0.));
#37424=DIRECTION('ref_axis',(1.,0.,0.));
#37425=DIRECTION('',(0.707106781186552,-0.707106781186543,-8.65956056235499E-17));
#37426=DIRECTION('center_axis',(0.,-1.,0.));
#37427=DIRECTION('ref_axis',(1.,0.,0.));
#37428=DIRECTION('',(0.707106781186552,0.707106781186543,8.65956056235499E-17));
#37429=DIRECTION('center_axis',(0.,1.,0.));
#37430=DIRECTION('ref_axis',(1.,0.,0.));
#37431=DIRECTION('',(0.707106781186552,-0.707106781186543,-8.65956056235499E-17));
#37432=DIRECTION('center_axis',(0.,-1.,0.));
#37433=DIRECTION('ref_axis',(1.,0.,0.));
#37434=DIRECTION('',(0.707106781186552,0.707106781186543,8.65956056235499E-17));
#37435=DIRECTION('center_axis',(0.,1.,0.));
#37436=DIRECTION('ref_axis',(1.,0.,0.));
#37437=DIRECTION('',(0.707106781186552,-0.707106781186543,-8.65956056235499E-17));
#37438=DIRECTION('center_axis',(0.,-1.,0.));
#37439=DIRECTION('ref_axis',(1.,0.,0.));
#37440=DIRECTION('',(0.707106781186552,0.707106781186543,8.65956056235499E-17));
#37441=DIRECTION('center_axis',(0.,1.,0.));
#37442=DIRECTION('ref_axis',(1.,0.,0.));
#37443=DIRECTION('',(0.707106781186552,-0.707106781186543,-8.65956056235499E-17));
#37444=DIRECTION('center_axis',(0.,-1.,0.));
#37445=DIRECTION('ref_axis',(1.,0.,0.));
#37446=DIRECTION('',(0.707106781186552,0.707106781186543,8.65956056235499E-17));
#37447=DIRECTION('center_axis',(0.,0.,-1.));
#37448=DIRECTION('ref_axis',(-0.707106781186546,-0.707106781186549,0.));
#37449=DIRECTION('',(-0.70710678118656,0.,-0.707106781186535));
#37450=DIRECTION('center_axis',(0.,0.,1.));
#37451=DIRECTION('ref_axis',(-0.707106781186546,-0.707106781186549,0.));
#37452=DIRECTION('',(0.,0.707106781186565,0.70710678118653));
#37453=DIRECTION('center_axis',(0.,0.,-1.));
#37454=DIRECTION('ref_axis',(-0.707106781186546,-0.707106781186549,0.));
#37455=DIRECTION('center_axis',(-0.707106781186522,0.,0.707106781186573));
#37456=DIRECTION('ref_axis',(0.707106781186573,0.,0.707106781186522));
#37457=DIRECTION('',(0.,1.,0.));
#37458=DIRECTION('',(-0.707106781186573,0.,-0.707106781186522));
#37459=DIRECTION('',(0.,-1.,0.));
#37460=DIRECTION('center_axis',(0.,0.,-1.));
#37461=DIRECTION('ref_axis',(-0.707106781186549,0.707106781186546,0.));
#37462=DIRECTION('',(0.,0.707106781186565,-0.70710678118653));
#37463=DIRECTION('center_axis',(0.,0.,1.));
#37464=DIRECTION('ref_axis',(-0.70710678118655,0.707106781186546,0.));
#37465=DIRECTION('center_axis',(0.,0.,-1.));
#37466=DIRECTION('ref_axis',(-0.707106781186549,0.707106781186546,0.));
#37467=DIRECTION('center_axis',(0.,0.707106781186527,0.707106781186568));
#37468=DIRECTION('ref_axis',(1.,0.,0.));
#37469=DIRECTION('',(1.,0.,0.));
#37470=DIRECTION('',(0.,0.707106781186568,-0.707106781186527));
#37471=DIRECTION('center_axis',(0.,0.,-1.));
#37472=DIRECTION('ref_axis',(0.707106781186546,0.707106781186549,0.));
#37473=DIRECTION('',(0.707106781186573,0.,-0.707106781186522));
#37474=DIRECTION('center_axis',(0.,0.,-1.));
#37475=DIRECTION('ref_axis',(0.707106781186546,0.707106781186549,0.));
#37476=DIRECTION('center_axis',(0.707106781186522,0.,0.707106781186573));
#37477=DIRECTION('ref_axis',(0.707106781186573,0.,-0.707106781186522));
#37478=DIRECTION('',(0.,-1.,0.));
#37479=DIRECTION('',(0.707106781186573,0.,-0.707106781186522));
#37480=DIRECTION('center_axis',(0.,0.,-1.));
#37481=DIRECTION('ref_axis',(0.707106781186546,-0.707106781186549,0.));
#37482=DIRECTION('',(0.,-0.707106781186579,-0.707106781186516));
#37483=DIRECTION('center_axis',(0.,0.,-1.));
#37484=DIRECTION('ref_axis',(0.707106781186546,-0.707106781186549,0.));
#37485=DIRECTION('center_axis',(0.,-0.707106781186527,0.707106781186568));
#37486=DIRECTION('ref_axis',(1.,0.,0.));
#37487=DIRECTION('',(-1.,0.,0.));
#37488=DIRECTION('center_axis',(0.,0.,1.));
#37489=DIRECTION('ref_axis',(-0.707106781186546,-0.707106781186549,0.));
#37490=DIRECTION('',(0.,0.,-1.));
#37491=DIRECTION('center_axis',(0.,0.,1.));
#37492=DIRECTION('ref_axis',(1.,0.,0.));
#37493=DIRECTION('center_axis',(0.,0.,1.));
#37494=DIRECTION('ref_axis',(-0.707106781186544,0.707106781186551,0.));
#37495=DIRECTION('',(-1.,0.,0.));
#37496=DIRECTION('center_axis',(0.,0.,1.));
#37497=DIRECTION('ref_axis',(0.707106781186544,0.707106781186551,0.));
#37498=DIRECTION('',(0.,1.,0.));
#37499=DIRECTION('center_axis',(0.,0.,1.));
#37500=DIRECTION('ref_axis',(0.707106781186544,-0.707106781186551,0.));
#37501=DIRECTION('',(1.,0.,0.));
#37502=DIRECTION('center_axis',(0.,0.,1.));
#37503=DIRECTION('ref_axis',(-0.707106781186553,-0.707106781186542,0.));
#37504=DIRECTION('',(0.,-1.,0.));
#37505=DIRECTION('center_axis',(0.,0.,1.));
#37506=DIRECTION('ref_axis',(-0.707106781186544,0.707106781186551,0.));
#37507=DIRECTION('',(0.707106781186585,0.,-0.70710678118651));
#37508=DIRECTION('center_axis',(0.,0.,-1.));
#37509=DIRECTION('ref_axis',(-0.707106781186544,0.707106781186551,0.));
#37510=DIRECTION('',(0.,0.707106781186566,0.707106781186529));
#37511=DIRECTION('center_axis',(0.707106781186522,0.,0.707106781186573));
#37512=DIRECTION('ref_axis',(0.707106781186573,0.,-0.707106781186522));
#37513=DIRECTION('',(0.707106781186573,0.,-0.707106781186522));
#37514=DIRECTION('',(0.,1.,0.));
#37515=DIRECTION('center_axis',(0.,0.,1.));
#37516=DIRECTION('ref_axis',(-0.707106781186553,-0.707106781186542,0.));
#37517=DIRECTION('',(0.,0.707106781186584,-0.707106781186511));
#37518=DIRECTION('center_axis',(0.,0.,-1.));
#37519=DIRECTION('ref_axis',(-0.707106781186553,-0.707106781186542,0.));
#37520=DIRECTION('center_axis',(0.,0.707106781186527,0.707106781186568));
#37521=DIRECTION('ref_axis',(1.,0.,0.));
#37522=DIRECTION('',(0.,0.707106781186568,-0.707106781186527));
#37523=DIRECTION('center_axis',(0.,0.,1.));
#37524=DIRECTION('ref_axis',(0.707106781186544,-0.707106781186551,0.));
#37525=DIRECTION('',(-0.707106781186598,0.,-0.707106781186497));
#37526=DIRECTION('center_axis',(-0.707106781186522,0.,0.707106781186573));
#37527=DIRECTION('ref_axis',(0.707106781186573,0.,0.707106781186522));
#37528=DIRECTION('',(-0.707106781186573,0.,-0.707106781186522));
#37529=DIRECTION('center_axis',(0.,0.,1.));
#37530=DIRECTION('ref_axis',(0.707106781186544,0.707106781186551,0.));
#37531=DIRECTION('',(0.,-0.707106781186579,-0.707106781186516));
#37532=DIRECTION('center_axis',(0.,-0.707106781186527,0.707106781186568));
#37533=DIRECTION('ref_axis',(1.,0.,0.));
#37534=DIRECTION('center_axis',(0.,0.,1.));
#37535=DIRECTION('ref_axis',(-0.707106781186544,0.707106781186551,0.));
#37536=DIRECTION('',(0.,0.,-1.));
#37537=DIRECTION('center_axis',(0.,0.,1.));
#37538=DIRECTION('ref_axis',(-0.707106781186553,-0.707106781186542,0.));
#37539=DIRECTION('',(0.,0.,1.));
#37540=DIRECTION('center_axis',(1.,0.,0.));
#37541=DIRECTION('ref_axis',(0.,1.,0.));
#37542=DIRECTION('center_axis',(-1.,0.,0.));
#37543=DIRECTION('ref_axis',(0.,-1.,0.));
#37544=DIRECTION('',(0.,0.,1.));
#37545=DIRECTION('center_axis',(0.,0.,1.));
#37546=DIRECTION('ref_axis',(-0.70710678118655,0.707106781186546,0.));
#70851=CARTESIAN_POINT('',(0.,0.,0.));
#70852=CARTESIAN_POINT('Origin',(30.,3.55,17.));
#70853=CARTESIAN_POINT('',(29.025,3.5,17.));
#70854=CARTESIAN_POINT('Origin',(30.,3.5,17.));
#70855=CARTESIAN_POINT('',(29.125,3.6,17.));
#70856=CARTESIAN_POINT('',(29.075,3.55,17.));
#70857=CARTESIAN_POINT('Origin',(30.,3.6,17.));
#70858=CARTESIAN_POINT('Origin',(26.5,3.5,1.));
#70859=CARTESIAN_POINT('',(33.2,3.5,1.1));
#70860=CARTESIAN_POINT('',(26.8,3.5,1.1));
#70861=CARTESIAN_POINT('',(28.25,3.5,1.1));
#70862=CARTESIAN_POINT('',(33.2,3.5,144.9));
#70863=CARTESIAN_POINT('',(33.2,3.5,1.));
#70864=CARTESIAN_POINT('',(26.8,3.5,144.9));
#70865=CARTESIAN_POINT('',(28.25,3.5,144.9));
#70866=CARTESIAN_POINT('',(26.8,3.5,1.));
#70867=CARTESIAN_POINT('',(29.025,3.5,6.));
#70868=CARTESIAN_POINT('Origin',(30.,3.5,6.));
#70869=CARTESIAN_POINT('',(29.025,3.5,137.5));
#70870=CARTESIAN_POINT('Origin',(30.,3.5,137.5));
#70871=CARTESIAN_POINT('',(28.6,3.5,83.75));
#70872=CARTESIAN_POINT('Origin',(30.,3.5,83.75));
#70873=CARTESIAN_POINT('',(28.6,3.5,74.75));
#70874=CARTESIAN_POINT('Origin',(30.,3.5,74.75));
#70875=CARTESIAN_POINT('',(28.6,3.5,56.75));
#70876=CARTESIAN_POINT('Origin',(30.,3.5,56.75));
#70877=CARTESIAN_POINT('',(28.6,3.5,38.75));
#70878=CARTESIAN_POINT('Origin',(30.,3.5,38.75));
#70879=CARTESIAN_POINT('',(28.6,3.5,65.75));
#70880=CARTESIAN_POINT('Origin',(30.,3.5,65.75));
#70881=CARTESIAN_POINT('',(28.6,3.5,47.75));
#70882=CARTESIAN_POINT('Origin',(30.,3.5,47.75));
#70883=CARTESIAN_POINT('',(29.025,3.5,33.5));
#70884=CARTESIAN_POINT('Origin',(30.,3.5,33.5));
#70885=CARTESIAN_POINT('',(29.025,3.5,142.5));
#70886=CARTESIAN_POINT('Origin',(30.,3.5,142.5));
#70887=CARTESIAN_POINT('Origin',(30.,0.,17.));
#70888=CARTESIAN_POINT('',(29.125,3.9,17.));
#70889=CARTESIAN_POINT('',(29.125,0.,17.));
#70890=CARTESIAN_POINT('Origin',(30.,3.9,17.));
#70891=CARTESIAN_POINT('Origin',(30.,3.55,6.));
#70892=CARTESIAN_POINT('',(29.125,3.6,6.));
#70893=CARTESIAN_POINT('',(29.075,3.55,6.));
#70894=CARTESIAN_POINT('Origin',(30.,3.6,6.));
#70895=CARTESIAN_POINT('Origin',(30.,0.,6.));
#70896=CARTESIAN_POINT('',(29.125,3.9,6.));
#70897=CARTESIAN_POINT('',(29.125,0.,6.));
#70898=CARTESIAN_POINT('Origin',(30.,3.9,6.));
#70899=CARTESIAN_POINT('Origin',(30.,3.55,142.5));
#70900=CARTESIAN_POINT('',(29.125,3.6,142.5));
#70901=CARTESIAN_POINT('',(29.075,3.55,142.5));
#70902=CARTESIAN_POINT('Origin',(30.,3.6,142.5));
#70903=CARTESIAN_POINT('Origin',(30.,0.,142.5));
#70904=CARTESIAN_POINT('',(29.125,3.9,142.5));
#70905=CARTESIAN_POINT('',(29.125,0.,142.5));
#70906=CARTESIAN_POINT('Origin',(30.,3.9,142.5));
#70907=CARTESIAN_POINT('Origin',(30.,3.55,137.5));
#70908=CARTESIAN_POINT('',(29.125,3.6,137.5));
#70909=CARTESIAN_POINT('',(29.075,3.55,137.5));
#70910=CARTESIAN_POINT('Origin',(30.,3.6,137.5));
#70911=CARTESIAN_POINT('Origin',(30.,0.,137.5));
#70912=CARTESIAN_POINT('',(29.125,3.9,137.5));
#70913=CARTESIAN_POINT('',(29.125,0.,137.5));
#70914=CARTESIAN_POINT('Origin',(30.,3.9,137.5));
#70915=CARTESIAN_POINT('Origin',(30.,3.55,33.5));
#70916=CARTESIAN_POINT('',(29.125,3.6,33.5));
#70917=CARTESIAN_POINT('',(29.075,3.55,33.5));
#70918=CARTESIAN_POINT('Origin',(30.,3.6,33.5));
#70919=CARTESIAN_POINT('Origin',(30.,0.,33.5));
#70920=CARTESIAN_POINT('',(29.125,3.9,33.5));
#70921=CARTESIAN_POINT('',(29.125,0.,33.5));
#70922=CARTESIAN_POINT('Origin',(30.,3.9,33.5));
#70923=CARTESIAN_POINT('Origin',(30.,3.55,83.75));
#70924=CARTESIAN_POINT('',(28.7,3.6,83.75));
#70925=CARTESIAN_POINT('',(28.65,3.55,83.75));
#70926=CARTESIAN_POINT('Origin',(30.,3.6,83.75));
#70927=CARTESIAN_POINT('Origin',(30.,0.,83.75));
#70928=CARTESIAN_POINT('',(28.7,3.9,83.75));
#70929=CARTESIAN_POINT('',(28.7,0.,83.75));
#70930=CARTESIAN_POINT('Origin',(30.,3.9,83.75));
#70931=CARTESIAN_POINT('Origin',(30.,3.55,47.75));
#70932=CARTESIAN_POINT('',(28.7,3.6,47.75));
#70933=CARTESIAN_POINT('',(28.65,3.55,47.75));
#70934=CARTESIAN_POINT('Origin',(30.,3.6,47.75));
#70935=CARTESIAN_POINT('Origin',(30.,0.,47.75));
#70936=CARTESIAN_POINT('',(28.7,3.9,47.75));
#70937=CARTESIAN_POINT('',(28.7,0.,47.75));
#70938=CARTESIAN_POINT('Origin',(30.,3.9,47.75));
#70939=CARTESIAN_POINT('Origin',(30.,-3.55,17.));
#70940=CARTESIAN_POINT('',(29.025,-3.5,17.));
#70941=CARTESIAN_POINT('Origin',(30.,-3.5,17.));
#70942=CARTESIAN_POINT('',(29.125,-3.6,17.));
#70943=CARTESIAN_POINT('',(29.075,-3.55,17.));
#70944=CARTESIAN_POINT('Origin',(30.,-3.6,17.));
#70945=CARTESIAN_POINT('Origin',(33.5,-3.5,1.));
#70946=CARTESIAN_POINT('',(26.8,-3.5,1.1));
#70947=CARTESIAN_POINT('',(33.2,-3.5,1.1));
#70948=CARTESIAN_POINT('',(31.75,-3.5,1.1));
#70949=CARTESIAN_POINT('',(26.8,-3.5,144.9));
#70950=CARTESIAN_POINT('',(26.8,-3.5,1.));
#70951=CARTESIAN_POINT('',(33.2,-3.5,144.9));
#70952=CARTESIAN_POINT('',(31.75,-3.5,144.9));
#70953=CARTESIAN_POINT('',(33.2,-3.5,1.));
#70954=CARTESIAN_POINT('',(29.025,-3.5,6.));
#70955=CARTESIAN_POINT('Origin',(30.,-3.5,6.));
#70956=CARTESIAN_POINT('',(29.025,-3.5,137.5));
#70957=CARTESIAN_POINT('Origin',(30.,-3.5,137.5));
#70958=CARTESIAN_POINT('',(28.6,-3.5,47.75));
#70959=CARTESIAN_POINT('Origin',(30.,-3.5,47.75));
#70960=CARTESIAN_POINT('',(28.6,-3.5,65.75));
#70961=CARTESIAN_POINT('Origin',(30.,-3.5,65.75));
#70962=CARTESIAN_POINT('',(28.6,-3.5,38.75));
#70963=CARTESIAN_POINT('Origin',(30.,-3.5,38.75));
#70964=CARTESIAN_POINT('',(28.6,-3.5,56.75));
#70965=CARTESIAN_POINT('Origin',(30.,-3.5,56.75));
#70966=CARTESIAN_POINT('',(28.6,-3.5,74.75));
#70967=CARTESIAN_POINT('Origin',(30.,-3.5,74.75));
#70968=CARTESIAN_POINT('',(28.6,-3.5,83.75));
#70969=CARTESIAN_POINT('Origin',(30.,-3.5,83.75));
#70970=CARTESIAN_POINT('',(29.025,-3.5,33.5));
#70971=CARTESIAN_POINT('Origin',(30.,-3.5,33.5));
#70972=CARTESIAN_POINT('',(29.025,-3.5,142.5));
#70973=CARTESIAN_POINT('Origin',(30.,-3.5,142.5));
#70974=CARTESIAN_POINT('Origin',(30.,0.,17.));
#70975=CARTESIAN_POINT('',(29.125,-3.9,17.));
#70976=CARTESIAN_POINT('Origin',(30.,-3.9,17.));
#70977=CARTESIAN_POINT('',(29.125,0.,17.));
#70978=CARTESIAN_POINT('Origin',(30.,-3.55,6.));
#70979=CARTESIAN_POINT('',(29.125,-3.6,6.));
#70980=CARTESIAN_POINT('',(29.075,-3.55,6.));
#70981=CARTESIAN_POINT('Origin',(30.,-3.6,6.));
#70982=CARTESIAN_POINT('Origin',(30.,0.,6.));
#70983=CARTESIAN_POINT('',(29.125,-3.9,6.));
#70984=CARTESIAN_POINT('Origin',(30.,-3.9,6.));
#70985=CARTESIAN_POINT('',(29.125,0.,6.));
#70986=CARTESIAN_POINT('Origin',(30.,-3.55,142.5));
#70987=CARTESIAN_POINT('',(29.125,-3.6,142.5));
#70988=CARTESIAN_POINT('',(29.075,-3.55,142.5));
#70989=CARTESIAN_POINT('Origin',(30.,-3.6,142.5));
#70990=CARTESIAN_POINT('Origin',(30.,0.,142.5));
#70991=CARTESIAN_POINT('',(29.125,-3.9,142.5));
#70992=CARTESIAN_POINT('Origin',(30.,-3.9,142.5));
#70993=CARTESIAN_POINT('',(29.125,0.,142.5));
#70994=CARTESIAN_POINT('Origin',(30.,-3.55,137.5));
#70995=CARTESIAN_POINT('',(29.125,-3.6,137.5));
#70996=CARTESIAN_POINT('',(29.075,-3.55,137.5));
#70997=CARTESIAN_POINT('Origin',(30.,-3.6,137.5));
#70998=CARTESIAN_POINT('Origin',(30.,0.,137.5));
#70999=CARTESIAN_POINT('',(29.125,-3.9,137.5));
#71000=CARTESIAN_POINT('Origin',(30.,-3.9,137.5));
#71001=CARTESIAN_POINT('',(29.125,0.,137.5));
#71002=CARTESIAN_POINT('Origin',(30.,-3.55,33.5));
#71003=CARTESIAN_POINT('',(29.125,-3.6,33.5));
#71004=CARTESIAN_POINT('',(29.075,-3.55,33.5));
#71005=CARTESIAN_POINT('Origin',(30.,-3.6,33.5));
#71006=CARTESIAN_POINT('Origin',(30.,0.,33.5));
#71007=CARTESIAN_POINT('',(29.125,-3.9,33.5));
#71008=CARTESIAN_POINT('Origin',(30.,-3.9,33.5));
#71009=CARTESIAN_POINT('',(29.125,0.,33.5));
#71010=CARTESIAN_POINT('Origin',(31.75,-3.55,1.05));
#71011=CARTESIAN_POINT('',(26.8,-3.6,1.));
#71012=CARTESIAN_POINT('',(26.8,-3.6,1.));
#71013=CARTESIAN_POINT('',(33.2,-3.6,1.));
#71014=CARTESIAN_POINT('',(33.2,-3.5,1.1));
#71015=CARTESIAN_POINT('',(31.75,-3.6,1.));
#71016=CARTESIAN_POINT('Origin',(26.8,-3.2,1.05));
#71017=CARTESIAN_POINT('',(26.4,-3.2,1.));
#71018=CARTESIAN_POINT('',(26.5,-3.2,1.1));
#71019=CARTESIAN_POINT('',(26.4,-3.2,1.));
#71020=CARTESIAN_POINT('Origin',(26.8,-3.2,1.1));
#71021=CARTESIAN_POINT('Origin',(26.8,-3.2,1.));
#71022=CARTESIAN_POINT('Origin',(26.45,-1.75,1.05));
#71023=CARTESIAN_POINT('',(26.4,3.2,1.));
#71024=CARTESIAN_POINT('',(26.5,3.2,1.1));
#71025=CARTESIAN_POINT('',(26.4,3.2,1.));
#71026=CARTESIAN_POINT('',(26.5,-1.75,1.1));
#71027=CARTESIAN_POINT('',(26.4,-1.75,1.));
#71028=CARTESIAN_POINT('Origin',(26.8,3.2,1.05));
#71029=CARTESIAN_POINT('',(26.8,3.6,1.));
#71030=CARTESIAN_POINT('',(26.8,3.6,1.));
#71031=CARTESIAN_POINT('Origin',(26.8,3.2,1.1));
#71032=CARTESIAN_POINT('Origin',(26.8,3.2,1.));
#71033=CARTESIAN_POINT('Origin',(28.25,3.55,1.05));
#71034=CARTESIAN_POINT('',(33.2,3.6,1.));
#71035=CARTESIAN_POINT('',(33.2,3.6,1.));
#71036=CARTESIAN_POINT('',(28.25,3.6,1.));
#71037=CARTESIAN_POINT('Origin',(33.2,3.2,1.05));
#71038=CARTESIAN_POINT('',(33.6,3.2,1.));
#71039=CARTESIAN_POINT('',(33.5,3.2,1.1));
#71040=CARTESIAN_POINT('',(33.6,3.2,1.));
#71041=CARTESIAN_POINT('Origin',(33.2,3.2,1.1));
#71042=CARTESIAN_POINT('Origin',(33.2,3.2,1.));
#71043=CARTESIAN_POINT('Origin',(33.55,1.75,1.05));
#71044=CARTESIAN_POINT('',(33.6,-3.2,1.));
#71045=CARTESIAN_POINT('',(33.5,-3.2,1.1));
#71046=CARTESIAN_POINT('',(33.6,-3.2,1.));
#71047=CARTESIAN_POINT('',(33.5,1.75,1.1));
#71048=CARTESIAN_POINT('',(33.6,1.75,1.));
#71049=CARTESIAN_POINT('Origin',(33.2,-3.2,1.05));
#71050=CARTESIAN_POINT('Origin',(33.2,-3.2,1.1));
#71051=CARTESIAN_POINT('Origin',(33.2,-3.2,1.));
#71052=CARTESIAN_POINT('Origin',(33.2,3.2,1.));
#71053=CARTESIAN_POINT('',(33.5,3.2,144.9));
#71054=CARTESIAN_POINT('',(33.5,3.2,1.));
#71055=CARTESIAN_POINT('Origin',(33.2,3.2,144.9));
#71056=CARTESIAN_POINT('Origin',(33.5,3.5,1.));
#71057=CARTESIAN_POINT('',(33.5,-3.2,144.9));
#71058=CARTESIAN_POINT('',(33.5,-3.2,1.));
#71059=CARTESIAN_POINT('',(33.5,1.75,144.9));
#71060=CARTESIAN_POINT('Origin',(33.2,-3.2,1.));
#71061=CARTESIAN_POINT('Origin',(33.2,-3.2,144.9));
#71062=CARTESIAN_POINT('Origin',(30.,0.,1.));
#71063=CARTESIAN_POINT('',(33.2,3.9,1.));
#71064=CARTESIAN_POINT('',(26.8,3.9,1.));
#71065=CARTESIAN_POINT('',(32.,3.9,1.));
#71066=CARTESIAN_POINT('',(33.9,3.2,1.));
#71067=CARTESIAN_POINT('Origin',(33.2,3.2,1.));
#71068=CARTESIAN_POINT('',(33.9,-3.2,1.));
#71069=CARTESIAN_POINT('',(33.9,-2.,1.));
#71070=CARTESIAN_POINT('',(33.2,-3.9,1.));
#71071=CARTESIAN_POINT('Origin',(33.2,-3.2,1.));
#71072=CARTESIAN_POINT('',(26.8,-3.9,1.));
#71073=CARTESIAN_POINT('',(28.,-3.9,1.));
#71074=CARTESIAN_POINT('',(26.1,-3.2,1.));
#71075=CARTESIAN_POINT('Origin',(26.8,-3.2,1.));
#71076=CARTESIAN_POINT('',(26.1,3.2,1.));
#71077=CARTESIAN_POINT('',(26.1,2.,1.));
#71078=CARTESIAN_POINT('Origin',(26.8,3.2,1.));
#71079=CARTESIAN_POINT('Origin',(30.,-3.55,83.75));
#71080=CARTESIAN_POINT('',(28.7,-3.6,83.75));
#71081=CARTESIAN_POINT('',(28.65,-3.55,83.75));
#71082=CARTESIAN_POINT('Origin',(30.,-3.6,83.75));
#71083=CARTESIAN_POINT('Origin',(30.,0.,83.75));
#71084=CARTESIAN_POINT('',(28.7,-3.9,83.75));
#71085=CARTESIAN_POINT('Origin',(30.,-3.9,83.75));
#71086=CARTESIAN_POINT('',(28.7,0.,83.75));
#71087=CARTESIAN_POINT('Origin',(30.,-3.55,47.75));
#71088=CARTESIAN_POINT('',(28.7,-3.6,47.75));
#71089=CARTESIAN_POINT('',(28.65,-3.55,47.75));
#71090=CARTESIAN_POINT('Origin',(30.,-3.6,47.75));
#71091=CARTESIAN_POINT('Origin',(30.,0.,47.75));
#71092=CARTESIAN_POINT('',(28.7,-3.9,47.75));
#71093=CARTESIAN_POINT('Origin',(30.,-3.9,47.75));
#71094=CARTESIAN_POINT('',(28.7,0.,47.75));
#71095=CARTESIAN_POINT('Origin',(30.,-3.55,74.75));
#71096=CARTESIAN_POINT('',(28.7,-3.6,74.75));
#71097=CARTESIAN_POINT('',(28.65,-3.55,74.75));
#71098=CARTESIAN_POINT('Origin',(30.,-3.6,74.75));
#71099=CARTESIAN_POINT('Origin',(30.,0.,74.75));
#71100=CARTESIAN_POINT('',(28.7,-3.9,74.75));
#71101=CARTESIAN_POINT('Origin',(30.,-3.9,74.75));
#71102=CARTESIAN_POINT('',(28.7,0.,74.75));
#71103=CARTESIAN_POINT('Origin',(30.,3.55,74.75));
#71104=CARTESIAN_POINT('',(28.7,3.6,74.75));
#71105=CARTESIAN_POINT('',(28.65,3.55,74.75));
#71106=CARTESIAN_POINT('Origin',(30.,3.6,74.75));
#71107=CARTESIAN_POINT('Origin',(30.,0.,74.75));
#71108=CARTESIAN_POINT('',(28.7,3.9,74.75));
#71109=CARTESIAN_POINT('',(28.7,0.,74.75));
#71110=CARTESIAN_POINT('Origin',(30.,3.9,74.75));
#71111=CARTESIAN_POINT('Origin',(30.,-3.55,65.75));
#71112=CARTESIAN_POINT('',(28.7,-3.6,65.75));
#71113=CARTESIAN_POINT('',(28.65,-3.55,65.75));
#71114=CARTESIAN_POINT('Origin',(30.,-3.6,65.75));
#71115=CARTESIAN_POINT('Origin',(30.,0.,65.75));
#71116=CARTESIAN_POINT('',(28.7,-3.9,65.75));
#71117=CARTESIAN_POINT('Origin',(30.,-3.9,65.75));
#71118=CARTESIAN_POINT('',(28.7,0.,65.75));
#71119=CARTESIAN_POINT('Origin',(30.,3.55,65.75));
#71120=CARTESIAN_POINT('',(28.7,3.6,65.75));
#71121=CARTESIAN_POINT('',(28.65,3.55,65.75));
#71122=CARTESIAN_POINT('Origin',(30.,3.6,65.75));
#71123=CARTESIAN_POINT('Origin',(30.,0.,65.75));
#71124=CARTESIAN_POINT('',(28.7,3.9,65.75));
#71125=CARTESIAN_POINT('',(28.7,0.,65.75));
#71126=CARTESIAN_POINT('Origin',(30.,3.9,65.75));
#71127=CARTESIAN_POINT('Origin',(30.,-3.55,56.75));
#71128=CARTESIAN_POINT('',(28.7,-3.6,56.75));
#71129=CARTESIAN_POINT('',(28.65,-3.55,56.75));
#71130=CARTESIAN_POINT('Origin',(30.,-3.6,56.75));
#71131=CARTESIAN_POINT('Origin',(30.,0.,56.75));
#71132=CARTESIAN_POINT('',(28.7,-3.9,56.75));
#71133=CARTESIAN_POINT('Origin',(30.,-3.9,56.75));
#71134=CARTESIAN_POINT('',(28.7,0.,56.75));
#71135=CARTESIAN_POINT('Origin',(30.,3.55,56.75));
#71136=CARTESIAN_POINT('',(28.7,3.6,56.75));
#71137=CARTESIAN_POINT('',(28.65,3.55,56.75));
#71138=CARTESIAN_POINT('Origin',(30.,3.6,56.75));
#71139=CARTESIAN_POINT('Origin',(30.,0.,56.75));
#71140=CARTESIAN_POINT('',(28.7,3.9,56.75));
#71141=CARTESIAN_POINT('',(28.7,0.,56.75));
#71142=CARTESIAN_POINT('Origin',(30.,3.9,56.75));
#71143=CARTESIAN_POINT('Origin',(30.,-3.55,38.75));
#71144=CARTESIAN_POINT('',(28.7,-3.6,38.75));
#71145=CARTESIAN_POINT('',(28.65,-3.55,38.75));
#71146=CARTESIAN_POINT('Origin',(30.,-3.6,38.75));
#71147=CARTESIAN_POINT('Origin',(30.,0.,38.75));
#71148=CARTESIAN_POINT('',(28.7,-3.9,38.75));
#71149=CARTESIAN_POINT('Origin',(30.,-3.9,38.75));
#71150=CARTESIAN_POINT('',(28.7,0.,38.75));
#71151=CARTESIAN_POINT('Origin',(30.,-3.95,17.));
#71152=CARTESIAN_POINT('',(29.025,-4.,17.));
#71153=CARTESIAN_POINT('Origin',(30.,-4.,17.));
#71154=CARTESIAN_POINT('',(29.075,-3.95,17.));
#71155=CARTESIAN_POINT('Origin',(26.,-4.,1.));
#71156=CARTESIAN_POINT('',(33.2,-4.,1.1));
#71157=CARTESIAN_POINT('',(26.8,-4.,1.1));
#71158=CARTESIAN_POINT('',(28.,-4.,1.1));
#71159=CARTESIAN_POINT('',(33.2,-4.,144.9));
#71160=CARTESIAN_POINT('',(33.2,-4.,1.));
#71161=CARTESIAN_POINT('',(26.8,-4.,144.9));
#71162=CARTESIAN_POINT('',(28.,-4.,144.9));
#71163=CARTESIAN_POINT('',(26.8,-4.,1.));
#71164=CARTESIAN_POINT('',(29.025,-4.,6.));
#71165=CARTESIAN_POINT('Origin',(30.,-4.,6.));
#71166=CARTESIAN_POINT('',(29.025,-4.,137.5));
#71167=CARTESIAN_POINT('Origin',(30.,-4.,137.5));
#71168=CARTESIAN_POINT('',(28.6,-4.,38.75));
#71169=CARTESIAN_POINT('Origin',(30.,-4.,38.75));
#71170=CARTESIAN_POINT('',(28.6,-4.,65.75));
#71171=CARTESIAN_POINT('Origin',(30.,-4.,65.75));
#71172=CARTESIAN_POINT('',(28.6,-4.,83.75));
#71173=CARTESIAN_POINT('Origin',(30.,-4.,83.75));
#71174=CARTESIAN_POINT('',(28.6,-4.,47.75));
#71175=CARTESIAN_POINT('Origin',(30.,-4.,47.75));
#71176=CARTESIAN_POINT('',(28.6,-4.,74.75));
#71177=CARTESIAN_POINT('Origin',(30.,-4.,74.75));
#71178=CARTESIAN_POINT('',(28.6,-4.,56.75));
#71179=CARTESIAN_POINT('Origin',(30.,-4.,56.75));
#71180=CARTESIAN_POINT('',(29.025,-4.,33.5));
#71181=CARTESIAN_POINT('Origin',(30.,-4.,33.5));
#71182=CARTESIAN_POINT('',(29.025,-4.,142.5));
#71183=CARTESIAN_POINT('Origin',(30.,-4.,142.5));
#71184=CARTESIAN_POINT('Origin',(30.,-3.95,6.));
#71185=CARTESIAN_POINT('',(29.075,-3.95,6.));
#71186=CARTESIAN_POINT('Origin',(30.,-3.95,142.5));
#71187=CARTESIAN_POINT('',(29.075,-3.95,142.5));
#71188=CARTESIAN_POINT('Origin',(30.,-3.95,137.5));
#71189=CARTESIAN_POINT('',(29.075,-3.95,137.5));
#71190=CARTESIAN_POINT('Origin',(30.,-3.95,33.5));
#71191=CARTESIAN_POINT('',(29.075,-3.95,33.5));
#71192=CARTESIAN_POINT('Origin',(30.,3.55,38.75));
#71193=CARTESIAN_POINT('',(28.7,3.6,38.75));
#71194=CARTESIAN_POINT('',(28.65,3.55,38.75));
#71195=CARTESIAN_POINT('Origin',(30.,3.6,38.75));
#71196=CARTESIAN_POINT('Origin',(30.,0.,38.75));
#71197=CARTESIAN_POINT('',(28.7,3.9,38.75));
#71198=CARTESIAN_POINT('',(28.7,0.,38.75));
#71199=CARTESIAN_POINT('Origin',(30.,3.9,38.75));
#71200=CARTESIAN_POINT('Origin',(30.,3.95,17.));
#71201=CARTESIAN_POINT('',(29.025,4.,17.));
#71202=CARTESIAN_POINT('Origin',(30.,4.,17.));
#71203=CARTESIAN_POINT('',(29.075,3.95,17.));
#71204=CARTESIAN_POINT('Origin',(34.,4.,1.));
#71205=CARTESIAN_POINT('',(26.8,4.,1.1));
#71206=CARTESIAN_POINT('',(33.2,4.,1.1));
#71207=CARTESIAN_POINT('',(32.,4.,1.1));
#71208=CARTESIAN_POINT('',(26.8,4.,144.9));
#71209=CARTESIAN_POINT('',(26.8,4.,1.));
#71210=CARTESIAN_POINT('',(33.2,4.,144.9));
#71211=CARTESIAN_POINT('',(32.,4.,144.9));
#71212=CARTESIAN_POINT('',(33.2,4.,1.));
#71213=CARTESIAN_POINT('',(29.025,4.,6.));
#71214=CARTESIAN_POINT('Origin',(30.,4.,6.));
#71215=CARTESIAN_POINT('',(29.025,4.,137.5));
#71216=CARTESIAN_POINT('Origin',(30.,4.,137.5));
#71217=CARTESIAN_POINT('',(28.6,4.,56.75));
#71218=CARTESIAN_POINT('Origin',(30.,4.,56.75));
#71219=CARTESIAN_POINT('',(28.6,4.,74.75));
#71220=CARTESIAN_POINT('Origin',(30.,4.,74.75));
#71221=CARTESIAN_POINT('',(28.6,4.,47.75));
#71222=CARTESIAN_POINT('Origin',(30.,4.,47.75));
#71223=CARTESIAN_POINT('',(28.6,4.,83.75));
#71224=CARTESIAN_POINT('Origin',(30.,4.,83.75));
#71225=CARTESIAN_POINT('',(28.6,4.,65.75));
#71226=CARTESIAN_POINT('Origin',(30.,4.,65.75));
#71227=CARTESIAN_POINT('',(28.6,4.,38.75));
#71228=CARTESIAN_POINT('Origin',(30.,4.,38.75));
#71229=CARTESIAN_POINT('',(29.025,4.,33.5));
#71230=CARTESIAN_POINT('Origin',(30.,4.,33.5));
#71231=CARTESIAN_POINT('',(29.025,4.,142.5));
#71232=CARTESIAN_POINT('Origin',(30.,4.,142.5));
#71233=CARTESIAN_POINT('Origin',(30.,3.95,6.));
#71234=CARTESIAN_POINT('',(29.075,3.95,6.));
#71235=CARTESIAN_POINT('Origin',(30.,3.95,142.5));
#71236=CARTESIAN_POINT('',(29.075,3.95,142.5));
#71237=CARTESIAN_POINT('Origin',(30.,3.95,137.5));
#71238=CARTESIAN_POINT('',(29.075,3.95,137.5));
#71239=CARTESIAN_POINT('Origin',(30.,3.95,33.5));
#71240=CARTESIAN_POINT('',(29.075,3.95,33.5));
#71241=CARTESIAN_POINT('Origin',(32.,3.95,1.05));
#71242=CARTESIAN_POINT('',(26.8,3.9,1.));
#71243=CARTESIAN_POINT('',(33.2,4.,1.1));
#71244=CARTESIAN_POINT('Origin',(26.8,3.2,1.05));
#71245=CARTESIAN_POINT('',(26.,3.2,1.1));
#71246=CARTESIAN_POINT('',(26.1,3.2,1.));
#71247=CARTESIAN_POINT('Origin',(26.8,3.2,1.1));
#71248=CARTESIAN_POINT('Origin',(26.05,2.,1.05));
#71249=CARTESIAN_POINT('',(26.,-3.2,1.1));
#71250=CARTESIAN_POINT('',(26.1,-3.2,1.));
#71251=CARTESIAN_POINT('',(26.,2.,1.1));
#71252=CARTESIAN_POINT('Origin',(26.8,-3.2,1.05));
#71253=CARTESIAN_POINT('',(26.8,-3.9,1.));
#71254=CARTESIAN_POINT('Origin',(26.8,-3.2,1.1));
#71255=CARTESIAN_POINT('Origin',(28.,-3.95,1.05));
#71256=CARTESIAN_POINT('',(33.2,-3.9,1.));
#71257=CARTESIAN_POINT('Origin',(33.2,-3.2,1.05));
#71258=CARTESIAN_POINT('',(34.,-3.2,1.1));
#71259=CARTESIAN_POINT('',(33.9,-3.2,1.));
#71260=CARTESIAN_POINT('Origin',(33.2,-3.2,1.1));
#71261=CARTESIAN_POINT('Origin',(33.95,-2.,1.05));
#71262=CARTESIAN_POINT('',(34.,3.2,1.1));
#71263=CARTESIAN_POINT('',(33.9,3.2,1.));
#71264=CARTESIAN_POINT('',(34.,-2.,1.1));
#71265=CARTESIAN_POINT('Origin',(33.2,3.2,1.05));
#71266=CARTESIAN_POINT('Origin',(33.2,3.2,1.1));
#71267=CARTESIAN_POINT('Origin',(33.2,-3.2,1.));
#71268=CARTESIAN_POINT('',(34.,-3.2,144.9));
#71269=CARTESIAN_POINT('',(34.,-3.2,1.));
#71270=CARTESIAN_POINT('Origin',(33.2,-3.2,144.9));
#71271=CARTESIAN_POINT('Origin',(34.,-4.,1.));
#71272=CARTESIAN_POINT('',(34.,3.2,144.9));
#71273=CARTESIAN_POINT('',(34.,3.2,1.));
#71274=CARTESIAN_POINT('',(34.,-2.,144.9));
#71275=CARTESIAN_POINT('Origin',(33.2,3.2,1.));
#71276=CARTESIAN_POINT('Origin',(33.2,3.2,144.9));
#71277=CARTESIAN_POINT('Origin',(30.,3.95,38.75));
#71278=CARTESIAN_POINT('',(28.65,3.95,38.75));
#71279=CARTESIAN_POINT('Origin',(30.,-3.95,38.75));
#71280=CARTESIAN_POINT('',(28.65,-3.95,38.75));
#71281=CARTESIAN_POINT('Origin',(30.,3.95,56.75));
#71282=CARTESIAN_POINT('',(28.65,3.95,56.75));
#71283=CARTESIAN_POINT('Origin',(30.,-3.95,56.75));
#71284=CARTESIAN_POINT('',(28.65,-3.95,56.75));
#71285=CARTESIAN_POINT('Origin',(30.,3.95,65.75));
#71286=CARTESIAN_POINT('',(28.65,3.95,65.75));
#71287=CARTESIAN_POINT('Origin',(30.,-3.95,65.75));
#71288=CARTESIAN_POINT('',(28.65,-3.95,65.75));
#71289=CARTESIAN_POINT('Origin',(30.,3.95,74.75));
#71290=CARTESIAN_POINT('',(28.65,3.95,74.75));
#71291=CARTESIAN_POINT('Origin',(30.,-3.95,74.75));
#71292=CARTESIAN_POINT('',(28.65,-3.95,74.75));
#71293=CARTESIAN_POINT('Origin',(30.,3.95,83.75));
#71294=CARTESIAN_POINT('',(28.65,3.95,83.75));
#71295=CARTESIAN_POINT('Origin',(30.,-3.95,83.75));
#71296=CARTESIAN_POINT('',(28.65,-3.95,83.75));
#71297=CARTESIAN_POINT('Origin',(30.,3.95,47.75));
#71298=CARTESIAN_POINT('',(28.65,3.95,47.75));
#71299=CARTESIAN_POINT('Origin',(30.,-3.95,47.75));
#71300=CARTESIAN_POINT('',(28.65,-3.95,47.75));
#71301=CARTESIAN_POINT('Origin',(26.8,-3.2,144.95));
#71302=CARTESIAN_POINT('',(26.1,-3.2,145.));
#71303=CARTESIAN_POINT('',(26.,-3.2,144.9));
#71304=CARTESIAN_POINT('',(26.1,-3.2,145.));
#71305=CARTESIAN_POINT('Origin',(26.8,-3.2,144.9));
#71306=CARTESIAN_POINT('',(26.8,-3.9,145.));
#71307=CARTESIAN_POINT('',(26.8,-4.,144.9));
#71308=CARTESIAN_POINT('Origin',(26.8,-3.2,145.));
#71309=CARTESIAN_POINT('Origin',(26.05,2.,144.95));
#71310=CARTESIAN_POINT('',(26.1,3.2,145.));
#71311=CARTESIAN_POINT('',(26.1,2.,145.));
#71312=CARTESIAN_POINT('',(26.,3.2,144.9));
#71313=CARTESIAN_POINT('',(26.1,3.2,145.));
#71314=CARTESIAN_POINT('',(26.,2.,144.9));
#71315=CARTESIAN_POINT('Origin',(26.8,3.2,144.95));
#71316=CARTESIAN_POINT('',(26.8,3.9,145.));
#71317=CARTESIAN_POINT('',(26.8,3.9,145.));
#71318=CARTESIAN_POINT('Origin',(26.8,3.2,144.9));
#71319=CARTESIAN_POINT('Origin',(26.8,3.2,145.));
#71320=CARTESIAN_POINT('Origin',(32.,3.95,144.95));
#71321=CARTESIAN_POINT('',(33.2,3.9,145.));
#71322=CARTESIAN_POINT('',(32.,3.9,145.));
#71323=CARTESIAN_POINT('',(33.2,3.9,145.));
#71324=CARTESIAN_POINT('Origin',(33.2,3.2,144.95));
#71325=CARTESIAN_POINT('',(33.9,3.2,145.));
#71326=CARTESIAN_POINT('',(33.9,3.2,145.));
#71327=CARTESIAN_POINT('Origin',(33.2,3.2,145.));
#71328=CARTESIAN_POINT('Origin',(33.95,-2.,144.95));
#71329=CARTESIAN_POINT('',(33.9,-3.2,145.));
#71330=CARTESIAN_POINT('',(33.9,-2.,145.));
#71331=CARTESIAN_POINT('',(33.9,-3.2,145.));
#71332=CARTESIAN_POINT('Origin',(33.2,-3.2,144.95));
#71333=CARTESIAN_POINT('',(33.2,-3.9,145.));
#71334=CARTESIAN_POINT('',(33.2,-3.9,145.));
#71335=CARTESIAN_POINT('Origin',(33.2,-3.2,145.));
#71336=CARTESIAN_POINT('Origin',(28.,-3.95,144.95));
#71337=CARTESIAN_POINT('',(28.,-3.9,145.));
#71338=CARTESIAN_POINT('Origin',(26.8,-3.2,1.));
#71339=CARTESIAN_POINT('',(26.,-3.2,1.));
#71340=CARTESIAN_POINT('Origin',(30.,0.,145.));
#71341=CARTESIAN_POINT('',(26.8,3.6,145.));
#71342=CARTESIAN_POINT('',(26.4,3.2,145.));
#71343=CARTESIAN_POINT('Origin',(26.8,3.2,145.));
#71344=CARTESIAN_POINT('',(33.2,3.6,145.));
#71345=CARTESIAN_POINT('',(28.25,3.6,145.));
#71346=CARTESIAN_POINT('',(33.6,3.2,145.));
#71347=CARTESIAN_POINT('Origin',(33.2,3.2,145.));
#71348=CARTESIAN_POINT('',(33.6,-3.2,145.));
#71349=CARTESIAN_POINT('',(33.6,1.75,145.));
#71350=CARTESIAN_POINT('',(33.2,-3.6,145.));
#71351=CARTESIAN_POINT('Origin',(33.2,-3.2,145.));
#71352=CARTESIAN_POINT('',(26.8,-3.6,145.));
#71353=CARTESIAN_POINT('',(31.75,-3.6,145.));
#71354=CARTESIAN_POINT('',(26.4,-3.2,145.));
#71355=CARTESIAN_POINT('Origin',(26.8,-3.2,145.));
#71356=CARTESIAN_POINT('',(26.4,-1.75,145.));
#71357=CARTESIAN_POINT('Origin',(26.8,3.2,144.95));
#71358=CARTESIAN_POINT('',(26.5,3.2,144.9));
#71359=CARTESIAN_POINT('',(26.4,3.2,145.));
#71360=CARTESIAN_POINT('Origin',(26.8,3.2,144.9));
#71361=CARTESIAN_POINT('',(26.8,3.5,144.9));
#71362=CARTESIAN_POINT('Origin',(26.45,-1.75,144.95));
#71363=CARTESIAN_POINT('',(26.5,-3.2,144.9));
#71364=CARTESIAN_POINT('',(26.4,-3.2,145.));
#71365=CARTESIAN_POINT('',(26.5,-1.75,144.9));
#71366=CARTESIAN_POINT('Origin',(26.8,-3.2,144.95));
#71367=CARTESIAN_POINT('',(26.8,-3.6,145.));
#71368=CARTESIAN_POINT('Origin',(26.8,-3.2,144.9));
#71369=CARTESIAN_POINT('Origin',(31.75,-3.55,144.95));
#71370=CARTESIAN_POINT('',(33.2,-3.6,145.));
#71371=CARTESIAN_POINT('Origin',(33.2,-3.2,144.95));
#71372=CARTESIAN_POINT('',(33.6,-3.2,145.));
#71373=CARTESIAN_POINT('Origin',(33.55,1.75,144.95));
#71374=CARTESIAN_POINT('',(33.6,3.2,145.));
#71375=CARTESIAN_POINT('Origin',(33.2,3.2,144.95));
#71376=CARTESIAN_POINT('',(33.2,3.6,145.));
#71377=CARTESIAN_POINT('Origin',(28.25,3.55,144.95));
#71378=CARTESIAN_POINT('Origin',(26.8,3.2,1.));
#71379=CARTESIAN_POINT('',(26.5,3.2,1.));
#71380=CARTESIAN_POINT('Origin',(26.8,-3.2,1.));
#71381=CARTESIAN_POINT('',(26.5,-3.2,1.));
#71382=CARTESIAN_POINT('Origin',(26.5,-3.5,1.));
#71383=CARTESIAN_POINT('Origin',(26.,4.,1.));
#71384=CARTESIAN_POINT('',(26.,3.2,1.));
#71385=CARTESIAN_POINT('Origin',(26.8,3.2,1.));
#71470=UNCERTAINTY_MEASURE_WITH_UNIT(LENGTH_MEASURE(0.001),#71493,
'DISTANCE_ACCURACY_VALUE',
'Maximum model space distance between geometric entities at asserted c
onnectivities');
#71471=UNCERTAINTY_MEASURE_WITH_UNIT(LENGTH_MEASURE(0.001),#71493,
'DISTANCE_ACCURACY_VALUE',
'Maximum model space distance between geometric entities at asserted c
onnectivities');
#71491=(
GEOMETRIC_REPRESENTATION_CONTEXT(3)
GLOBAL_UNCERTAINTY_ASSIGNED_CONTEXT((#71470))
GLOBAL_UNIT_ASSIGNED_CONTEXT((#71493,#71495,#71496))
REPRESENTATION_CONTEXT('','3D')
);
#71492=(
GEOMETRIC_REPRESENTATION_CONTEXT(3)
GLOBAL_UNCERTAINTY_ASSIGNED_CONTEXT((#71471))
GLOBAL_UNIT_ASSIGNED_CONTEXT((#71493,#71495,#71496))
REPRESENTATION_CONTEXT('','3D')
);
#71493=(
LENGTH_UNIT()
NAMED_UNIT(*)
SI_UNIT(.CENTI.,.METRE.)
);
#71495=(
NAMED_UNIT(*)
PLANE_ANGLE_UNIT()
SI_UNIT($,.RADIAN.)
);
#71496=(
NAMED_UNIT(*)
SI_UNIT($,.STERADIAN.)
SOLID_ANGLE_UNIT()
);
#71516=SHAPE_DEFINITION_REPRESENTATION(#71536,#71621);
#71536=PRODUCT_DEFINITION_SHAPE('',$,#71642);
#71621=SHAPE_REPRESENTATION('',(#30553),#71491);
#71622=PRODUCT_DEFINITION_CONTEXT('part definition',#71684,'design');
#71642=PRODUCT_DEFINITION('2026-10-19-03-21-44-299',
'01_Upright_Column_L1440_RHS80x80x5',#71662,#71622);
#71662=PRODUCT_DEFINITION_FORMATION('',$,#71705);
#71684=APPLICATION_CONTEXT(
'Core Data for Automotive Mechanical Design Process');
#71685=PRODUCT_CONTEXT('part definition',#71684,'mechanical');
#71705=PRODUCT('2026-10-19-03-21-44-299',
'01_Upright_Column_L1440_RHS80x80x5',$,(#71685));
#71867=COLOUR_RGB('Light Blue',0.38,0.62,0.78);
#71868=FILL_AREA_STYLE_COLOUR('',#71867);
#71869=FILL_AREA_STYLE('',(#71868));
#71870=SURFACE_STYLE_FILL_AREA(#71869);
#71871=SURFACE_SIDE_STYLE('',(#71870));
#71872=SURFACE_STYLE_USAGE(.BOTH.,#71871);
#71873=PRESENTATION_STYLE_ASSIGNMENT((#71872));
ENDSEC;
END-ISO-10303-21;
